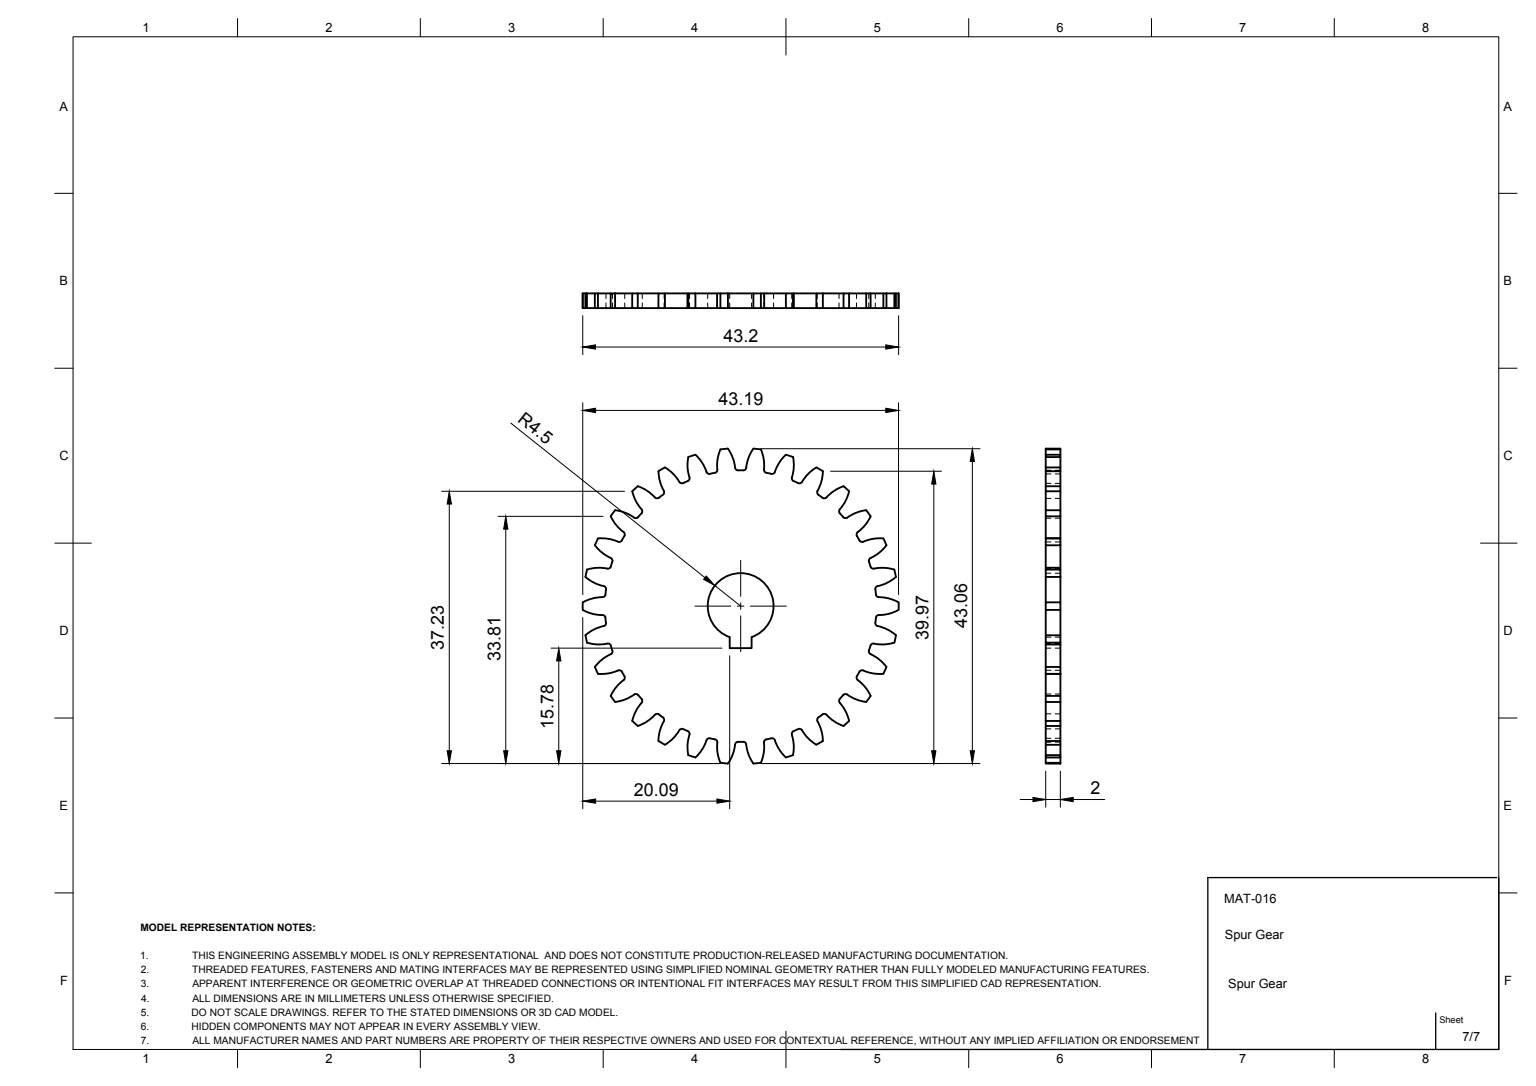
ISO-10303-21;
HEADER;
/* Generated by software containing ST-Developer
 * from STEP Tools, Inc. (www.steptools.com) 
 */

FILE_DESCRIPTION(
/* description */ ('STEP AP214'),
/* implementation_level */ '2;1');

FILE_NAME(
/* name */ 'Spur Gear.step',
/* time_stamp */ '2026-11-14T06:10:26-08:00',
/* author */ (''),
/* organization */ (''),
/* preprocessor_version */ 'ST-DEVELOPER v20.2',
/* originating_system */ 'Autodesk Translation Framework v15.17.0.0',
/* authorisation */ '');

FILE_SCHEMA (('AUTOMOTIVE_DESIGN { 1 0 10303 214 3 1 1 }'));
ENDSEC;

DATA;
#10=MECHANICAL_DESIGN_GEOMETRIC_PRESENTATION_REPRESENTATION('',(#166),#10413);
#150=SHAPE_REPRESENTATION_RELATIONSHIP('SRR','None',#10455,#158);
#158=ADVANCED_BREP_SHAPE_REPRESENTATION('',(#174),#10407);
#166=STYLED_ITEM('',(#10502),#174);
#174=MANIFOLD_SOLID_BREP('Body1',#5301);
#199=FACE_BOUND('',#668,.T.);
#200=FACE_BOUND('',#670,.T.);
#240=PLANE('',#5611);
#241=PLANE('',#5745);
#242=PLANE('',#6012);
#243=PLANE('',#6013);
#244=PLANE('',#6014);
#310=FACE_OUTER_BOUND('',#619,.T.);
#311=FACE_OUTER_BOUND('',#620,.T.);
#312=FACE_OUTER_BOUND('',#621,.T.);
#313=FACE_OUTER_BOUND('',#622,.T.);
#314=FACE_OUTER_BOUND('',#623,.T.);
#315=FACE_OUTER_BOUND('',#624,.T.);
#316=FACE_OUTER_BOUND('',#625,.T.);
#317=FACE_OUTER_BOUND('',#626,.T.);
#318=FACE_OUTER_BOUND('',#627,.T.);
#319=FACE_OUTER_BOUND('',#628,.T.);
#320=FACE_OUTER_BOUND('',#629,.T.);
#321=FACE_OUTER_BOUND('',#630,.T.);
#322=FACE_OUTER_BOUND('',#631,.T.);
#323=FACE_OUTER_BOUND('',#632,.T.);
#324=FACE_OUTER_BOUND('',#633,.T.);
#325=FACE_OUTER_BOUND('',#634,.T.);
#326=FACE_OUTER_BOUND('',#635,.T.);
#327=FACE_OUTER_BOUND('',#636,.T.);
#328=FACE_OUTER_BOUND('',#637,.T.);
#329=FACE_OUTER_BOUND('',#638,.T.);
#330=FACE_OUTER_BOUND('',#639,.T.);
#331=FACE_OUTER_BOUND('',#640,.T.);
#332=FACE_OUTER_BOUND('',#641,.T.);
#333=FACE_OUTER_BOUND('',#642,.T.);
#334=FACE_OUTER_BOUND('',#643,.T.);
#335=FACE_OUTER_BOUND('',#644,.T.);
#336=FACE_OUTER_BOUND('',#645,.T.);
#337=FACE_OUTER_BOUND('',#646,.T.);
#338=FACE_OUTER_BOUND('',#647,.T.);
#339=FACE_OUTER_BOUND('',#648,.T.);
#340=FACE_OUTER_BOUND('',#649,.T.);
#341=FACE_OUTER_BOUND('',#650,.T.);
#342=FACE_OUTER_BOUND('',#651,.T.);
#343=FACE_OUTER_BOUND('',#652,.T.);
#344=FACE_OUTER_BOUND('',#653,.T.);
#345=FACE_OUTER_BOUND('',#654,.T.);
#346=FACE_OUTER_BOUND('',#655,.T.);
#347=FACE_OUTER_BOUND('',#656,.T.);
#348=FACE_OUTER_BOUND('',#657,.T.);
#349=FACE_OUTER_BOUND('',#658,.T.);
#350=FACE_OUTER_BOUND('',#659,.T.);
#351=FACE_OUTER_BOUND('',#660,.T.);
#352=FACE_OUTER_BOUND('',#661,.T.);
#353=FACE_OUTER_BOUND('',#662,.T.);
#354=FACE_OUTER_BOUND('',#663,.T.);
#355=FACE_OUTER_BOUND('',#664,.T.);
#356=FACE_OUTER_BOUND('',#665,.T.);
#357=FACE_OUTER_BOUND('',#666,.T.);
#358=FACE_OUTER_BOUND('',#667,.T.);
#359=FACE_OUTER_BOUND('',#669,.T.);
#360=FACE_OUTER_BOUND('',#671,.T.);
#361=FACE_OUTER_BOUND('',#672,.T.);
#362=FACE_OUTER_BOUND('',#673,.T.);
#363=FACE_OUTER_BOUND('',#674,.T.);
#364=FACE_OUTER_BOUND('',#675,.T.);
#365=FACE_OUTER_BOUND('',#676,.T.);
#366=FACE_OUTER_BOUND('',#677,.T.);
#367=FACE_OUTER_BOUND('',#678,.T.);
#368=FACE_OUTER_BOUND('',#679,.T.);
#369=FACE_OUTER_BOUND('',#680,.T.);
#370=FACE_OUTER_BOUND('',#681,.T.);
#371=FACE_OUTER_BOUND('',#682,.T.);
#372=FACE_OUTER_BOUND('',#683,.T.);
#373=FACE_OUTER_BOUND('',#684,.T.);
#374=FACE_OUTER_BOUND('',#685,.T.);
#375=FACE_OUTER_BOUND('',#686,.T.);
#376=FACE_OUTER_BOUND('',#687,.T.);
#377=FACE_OUTER_BOUND('',#688,.T.);
#378=FACE_OUTER_BOUND('',#689,.T.);
#379=FACE_OUTER_BOUND('',#690,.T.);
#380=FACE_OUTER_BOUND('',#691,.T.);
#381=FACE_OUTER_BOUND('',#692,.T.);
#382=FACE_OUTER_BOUND('',#693,.T.);
#383=FACE_OUTER_BOUND('',#694,.T.);
#384=FACE_OUTER_BOUND('',#695,.T.);
#385=FACE_OUTER_BOUND('',#696,.T.);
#386=FACE_OUTER_BOUND('',#697,.T.);
#387=FACE_OUTER_BOUND('',#698,.T.);
#388=FACE_OUTER_BOUND('',#699,.T.);
#389=FACE_OUTER_BOUND('',#700,.T.);
#390=FACE_OUTER_BOUND('',#701,.T.);
#391=FACE_OUTER_BOUND('',#702,.T.);
#392=FACE_OUTER_BOUND('',#703,.T.);
#393=FACE_OUTER_BOUND('',#704,.T.);
#394=FACE_OUTER_BOUND('',#705,.T.);
#395=FACE_OUTER_BOUND('',#706,.T.);
#396=FACE_OUTER_BOUND('',#707,.T.);
#397=FACE_OUTER_BOUND('',#708,.T.);
#398=FACE_OUTER_BOUND('',#709,.T.);
#399=FACE_OUTER_BOUND('',#710,.T.);
#400=FACE_OUTER_BOUND('',#711,.T.);
#401=FACE_OUTER_BOUND('',#712,.T.);
#402=FACE_OUTER_BOUND('',#713,.T.);
#403=FACE_OUTER_BOUND('',#714,.T.);
#404=FACE_OUTER_BOUND('',#715,.T.);
#405=FACE_OUTER_BOUND('',#716,.T.);
#406=FACE_OUTER_BOUND('',#717,.T.);
#407=FACE_OUTER_BOUND('',#718,.T.);
#408=FACE_OUTER_BOUND('',#719,.T.);
#409=FACE_OUTER_BOUND('',#720,.T.);
#410=FACE_OUTER_BOUND('',#721,.T.);
#411=FACE_OUTER_BOUND('',#722,.T.);
#412=FACE_OUTER_BOUND('',#723,.T.);
#413=FACE_OUTER_BOUND('',#724,.T.);
#414=FACE_OUTER_BOUND('',#725,.T.);
#415=FACE_OUTER_BOUND('',#726,.T.);
#416=FACE_OUTER_BOUND('',#727,.T.);
#417=FACE_OUTER_BOUND('',#728,.T.);
#418=FACE_OUTER_BOUND('',#729,.T.);
#419=FACE_OUTER_BOUND('',#730,.T.);
#420=FACE_OUTER_BOUND('',#731,.T.);
#421=FACE_OUTER_BOUND('',#732,.T.);
#422=FACE_OUTER_BOUND('',#733,.T.);
#423=FACE_OUTER_BOUND('',#734,.T.);
#424=FACE_OUTER_BOUND('',#735,.T.);
#425=FACE_OUTER_BOUND('',#736,.T.);
#426=FACE_OUTER_BOUND('',#737,.T.);
#427=FACE_OUTER_BOUND('',#738,.T.);
#428=FACE_OUTER_BOUND('',#739,.T.);
#429=FACE_OUTER_BOUND('',#740,.T.);
#430=FACE_OUTER_BOUND('',#741,.T.);
#431=FACE_OUTER_BOUND('',#742,.T.);
#432=FACE_OUTER_BOUND('',#743,.T.);
#433=FACE_OUTER_BOUND('',#744,.T.);
#434=FACE_OUTER_BOUND('',#745,.T.);
#435=FACE_OUTER_BOUND('',#746,.T.);
#436=FACE_OUTER_BOUND('',#747,.T.);
#437=FACE_OUTER_BOUND('',#748,.T.);
#438=FACE_OUTER_BOUND('',#749,.T.);
#439=FACE_OUTER_BOUND('',#750,.T.);
#440=FACE_OUTER_BOUND('',#751,.T.);
#441=FACE_OUTER_BOUND('',#752,.T.);
#442=FACE_OUTER_BOUND('',#753,.T.);
#443=FACE_OUTER_BOUND('',#754,.T.);
#444=FACE_OUTER_BOUND('',#755,.T.);
#445=FACE_OUTER_BOUND('',#756,.T.);
#446=FACE_OUTER_BOUND('',#757,.T.);
#447=FACE_OUTER_BOUND('',#758,.T.);
#448=FACE_OUTER_BOUND('',#759,.T.);
#449=FACE_OUTER_BOUND('',#760,.T.);
#450=FACE_OUTER_BOUND('',#761,.T.);
#451=FACE_OUTER_BOUND('',#762,.T.);
#452=FACE_OUTER_BOUND('',#763,.T.);
#453=FACE_OUTER_BOUND('',#764,.T.);
#454=FACE_OUTER_BOUND('',#765,.T.);
#455=FACE_OUTER_BOUND('',#766,.T.);
#456=FACE_OUTER_BOUND('',#767,.T.);
#457=FACE_OUTER_BOUND('',#768,.T.);
#458=FACE_OUTER_BOUND('',#769,.T.);
#459=FACE_OUTER_BOUND('',#770,.T.);
#460=FACE_OUTER_BOUND('',#771,.T.);
#461=FACE_OUTER_BOUND('',#772,.T.);
#462=FACE_OUTER_BOUND('',#773,.T.);
#463=FACE_OUTER_BOUND('',#774,.T.);
#464=FACE_OUTER_BOUND('',#775,.T.);
#465=FACE_OUTER_BOUND('',#776,.T.);
#466=FACE_OUTER_BOUND('',#777,.T.);
#467=FACE_OUTER_BOUND('',#778,.T.);
#468=FACE_OUTER_BOUND('',#779,.T.);
#469=FACE_OUTER_BOUND('',#780,.T.);
#470=FACE_OUTER_BOUND('',#781,.T.);
#471=FACE_OUTER_BOUND('',#782,.T.);
#472=FACE_OUTER_BOUND('',#783,.T.);
#473=FACE_OUTER_BOUND('',#784,.T.);
#474=FACE_OUTER_BOUND('',#785,.T.);
#475=FACE_OUTER_BOUND('',#786,.T.);
#476=FACE_OUTER_BOUND('',#787,.T.);
#477=FACE_OUTER_BOUND('',#788,.T.);
#478=FACE_OUTER_BOUND('',#789,.T.);
#479=FACE_OUTER_BOUND('',#790,.T.);
#480=FACE_OUTER_BOUND('',#791,.T.);
#481=FACE_OUTER_BOUND('',#792,.T.);
#482=FACE_OUTER_BOUND('',#793,.T.);
#483=FACE_OUTER_BOUND('',#794,.T.);
#484=FACE_OUTER_BOUND('',#795,.T.);
#485=FACE_OUTER_BOUND('',#796,.T.);
#486=FACE_OUTER_BOUND('',#797,.T.);
#487=FACE_OUTER_BOUND('',#798,.T.);
#488=FACE_OUTER_BOUND('',#799,.T.);
#489=FACE_OUTER_BOUND('',#800,.T.);
#490=FACE_OUTER_BOUND('',#801,.T.);
#491=FACE_OUTER_BOUND('',#802,.T.);
#492=FACE_OUTER_BOUND('',#803,.T.);
#493=FACE_OUTER_BOUND('',#804,.T.);
#494=FACE_OUTER_BOUND('',#805,.T.);
#495=FACE_OUTER_BOUND('',#806,.T.);
#619=EDGE_LOOP('',(#3374,#3375,#3376,#3377));
#620=EDGE_LOOP('',(#3378,#3379,#3380,#3381));
#621=EDGE_LOOP('',(#3382,#3383,#3384,#3385));
#622=EDGE_LOOP('',(#3386,#3387,#3388,#3389));
#623=EDGE_LOOP('',(#3390,#3391,#3392,#3393));
#624=EDGE_LOOP('',(#3394,#3395,#3396,#3397));
#625=EDGE_LOOP('',(#3398,#3399,#3400,#3401));
#626=EDGE_LOOP('',(#3402,#3403,#3404,#3405));
#627=EDGE_LOOP('',(#3406,#3407,#3408,#3409));
#628=EDGE_LOOP('',(#3410,#3411,#3412,#3413));
#629=EDGE_LOOP('',(#3414,#3415,#3416,#3417));
#630=EDGE_LOOP('',(#3418,#3419,#3420,#3421));
#631=EDGE_LOOP('',(#3422,#3423,#3424,#3425));
#632=EDGE_LOOP('',(#3426,#3427,#3428,#3429));
#633=EDGE_LOOP('',(#3430,#3431,#3432,#3433));
#634=EDGE_LOOP('',(#3434,#3435,#3436,#3437));
#635=EDGE_LOOP('',(#3438,#3439,#3440,#3441));
#636=EDGE_LOOP('',(#3442,#3443,#3444,#3445));
#637=EDGE_LOOP('',(#3446,#3447,#3448,#3449));
#638=EDGE_LOOP('',(#3450,#3451,#3452,#3453));
#639=EDGE_LOOP('',(#3454,#3455,#3456,#3457));
#640=EDGE_LOOP('',(#3458,#3459,#3460,#3461));
#641=EDGE_LOOP('',(#3462,#3463,#3464,#3465));
#642=EDGE_LOOP('',(#3466,#3467,#3468,#3469));
#643=EDGE_LOOP('',(#3470,#3471,#3472,#3473));
#644=EDGE_LOOP('',(#3474,#3475,#3476,#3477));
#645=EDGE_LOOP('',(#3478,#3479,#3480,#3481));
#646=EDGE_LOOP('',(#3482,#3483,#3484,#3485));
#647=EDGE_LOOP('',(#3486,#3487,#3488,#3489));
#648=EDGE_LOOP('',(#3490,#3491,#3492,#3493));
#649=EDGE_LOOP('',(#3494,#3495,#3496,#3497));
#650=EDGE_LOOP('',(#3498,#3499,#3500,#3501));
#651=EDGE_LOOP('',(#3502,#3503,#3504,#3505));
#652=EDGE_LOOP('',(#3506,#3507,#3508,#3509));
#653=EDGE_LOOP('',(#3510,#3511,#3512,#3513));
#654=EDGE_LOOP('',(#3514,#3515,#3516,#3517));
#655=EDGE_LOOP('',(#3518,#3519,#3520,#3521));
#656=EDGE_LOOP('',(#3522,#3523,#3524,#3525));
#657=EDGE_LOOP('',(#3526,#3527,#3528,#3529));
#658=EDGE_LOOP('',(#3530,#3531,#3532,#3533));
#659=EDGE_LOOP('',(#3534,#3535,#3536,#3537));
#660=EDGE_LOOP('',(#3538,#3539,#3540,#3541));
#661=EDGE_LOOP('',(#3542,#3543,#3544,#3545));
#662=EDGE_LOOP('',(#3546,#3547,#3548,#3549));
#663=EDGE_LOOP('',(#3550,#3551,#3552,#3553));
#664=EDGE_LOOP('',(#3554,#3555,#3556,#3557));
#665=EDGE_LOOP('',(#3558,#3559,#3560,#3561));
#666=EDGE_LOOP('',(#3562,#3563,#3564,#3565));
#667=EDGE_LOOP('',(#3566,#3567,#3568,#3569,#3570,#3571,#3572,#3573,#3574,
#3575,#3576,#3577,#3578,#3579,#3580,#3581,#3582,#3583,#3584,#3585,#3586,
#3587,#3588,#3589,#3590,#3591,#3592,#3593,#3594,#3595,#3596,#3597,#3598,
#3599,#3600,#3601,#3602,#3603,#3604,#3605,#3606,#3607,#3608,#3609,#3610,
#3611,#3612,#3613,#3614,#3615,#3616,#3617,#3618,#3619,#3620,#3621,#3622,
#3623,#3624,#3625,#3626,#3627,#3628,#3629,#3630,#3631,#3632,#3633,#3634,
#3635,#3636,#3637,#3638,#3639,#3640,#3641,#3642,#3643,#3644,#3645,#3646,
#3647,#3648,#3649,#3650,#3651,#3652,#3653,#3654,#3655,#3656,#3657,#3658,
#3659,#3660,#3661,#3662,#3663,#3664,#3665,#3666,#3667,#3668,#3669,#3670,
#3671,#3672,#3673,#3674,#3675,#3676,#3677,#3678,#3679,#3680,#3681,#3682,
#3683,#3684,#3685,#3686,#3687,#3688,#3689,#3690,#3691,#3692,#3693,#3694,
#3695,#3696,#3697,#3698,#3699,#3700,#3701,#3702,#3703,#3704,#3705,#3706,
#3707,#3708,#3709,#3710,#3711,#3712,#3713,#3714,#3715,#3716,#3717,#3718,
#3719,#3720,#3721,#3722,#3723,#3724,#3725,#3726,#3727,#3728,#3729,#3730,
#3731,#3732,#3733,#3734,#3735,#3736,#3737,#3738,#3739,#3740,#3741,#3742,
#3743,#3744,#3745));
#668=EDGE_LOOP('',(#3746,#3747,#3748,#3749));
#669=EDGE_LOOP('',(#3750,#3751,#3752,#3753,#3754,#3755,#3756,#3757,#3758,
#3759,#3760,#3761,#3762,#3763,#3764,#3765,#3766,#3767,#3768,#3769,#3770,
#3771,#3772,#3773,#3774,#3775,#3776,#3777,#3778,#3779,#3780,#3781,#3782,
#3783,#3784,#3785,#3786,#3787,#3788,#3789,#3790,#3791,#3792,#3793,#3794,
#3795,#3796,#3797,#3798,#3799,#3800,#3801,#3802,#3803,#3804,#3805,#3806,
#3807,#3808,#3809,#3810,#3811,#3812,#3813,#3814,#3815,#3816,#3817,#3818,
#3819,#3820,#3821,#3822,#3823,#3824,#3825,#3826,#3827,#3828,#3829,#3830,
#3831,#3832,#3833,#3834,#3835,#3836,#3837,#3838,#3839,#3840,#3841,#3842,
#3843,#3844,#3845,#3846,#3847,#3848,#3849,#3850,#3851,#3852,#3853,#3854,
#3855,#3856,#3857,#3858,#3859,#3860,#3861,#3862,#3863,#3864,#3865,#3866,
#3867,#3868,#3869,#3870,#3871,#3872,#3873,#3874,#3875,#3876,#3877,#3878,
#3879,#3880,#3881,#3882,#3883,#3884,#3885,#3886,#3887,#3888,#3889,#3890,
#3891,#3892,#3893,#3894,#3895,#3896,#3897,#3898,#3899,#3900,#3901,#3902,
#3903,#3904,#3905,#3906,#3907,#3908,#3909,#3910,#3911,#3912,#3913,#3914,
#3915,#3916,#3917,#3918,#3919,#3920,#3921,#3922,#3923,#3924,#3925,#3926,
#3927,#3928,#3929));
#670=EDGE_LOOP('',(#3930,#3931,#3932,#3933));
#671=EDGE_LOOP('',(#3934,#3935,#3936,#3937));
#672=EDGE_LOOP('',(#3938,#3939,#3940,#3941));
#673=EDGE_LOOP('',(#3942,#3943,#3944,#3945));
#674=EDGE_LOOP('',(#3946,#3947,#3948,#3949));
#675=EDGE_LOOP('',(#3950,#3951,#3952,#3953));
#676=EDGE_LOOP('',(#3954,#3955,#3956,#3957));
#677=EDGE_LOOP('',(#3958,#3959,#3960,#3961));
#678=EDGE_LOOP('',(#3962,#3963,#3964,#3965));
#679=EDGE_LOOP('',(#3966,#3967,#3968,#3969));
#680=EDGE_LOOP('',(#3970,#3971,#3972,#3973));
#681=EDGE_LOOP('',(#3974,#3975,#3976,#3977));
#682=EDGE_LOOP('',(#3978,#3979,#3980,#3981));
#683=EDGE_LOOP('',(#3982,#3983,#3984,#3985));
#684=EDGE_LOOP('',(#3986,#3987,#3988,#3989));
#685=EDGE_LOOP('',(#3990,#3991,#3992,#3993));
#686=EDGE_LOOP('',(#3994,#3995,#3996,#3997));
#687=EDGE_LOOP('',(#3998,#3999,#4000,#4001));
#688=EDGE_LOOP('',(#4002,#4003,#4004,#4005));
#689=EDGE_LOOP('',(#4006,#4007,#4008,#4009));
#690=EDGE_LOOP('',(#4010,#4011,#4012,#4013));
#691=EDGE_LOOP('',(#4014,#4015,#4016,#4017));
#692=EDGE_LOOP('',(#4018,#4019,#4020,#4021));
#693=EDGE_LOOP('',(#4022,#4023,#4024,#4025));
#694=EDGE_LOOP('',(#4026,#4027,#4028,#4029));
#695=EDGE_LOOP('',(#4030,#4031,#4032,#4033));
#696=EDGE_LOOP('',(#4034,#4035,#4036,#4037));
#697=EDGE_LOOP('',(#4038,#4039,#4040,#4041));
#698=EDGE_LOOP('',(#4042,#4043,#4044,#4045));
#699=EDGE_LOOP('',(#4046,#4047,#4048,#4049));
#700=EDGE_LOOP('',(#4050,#4051,#4052,#4053));
#701=EDGE_LOOP('',(#4054,#4055,#4056,#4057));
#702=EDGE_LOOP('',(#4058,#4059,#4060,#4061));
#703=EDGE_LOOP('',(#4062,#4063,#4064,#4065));
#704=EDGE_LOOP('',(#4066,#4067,#4068,#4069));
#705=EDGE_LOOP('',(#4070,#4071,#4072,#4073));
#706=EDGE_LOOP('',(#4074,#4075,#4076,#4077));
#707=EDGE_LOOP('',(#4078,#4079,#4080,#4081));
#708=EDGE_LOOP('',(#4082,#4083,#4084,#4085));
#709=EDGE_LOOP('',(#4086,#4087,#4088,#4089));
#710=EDGE_LOOP('',(#4090,#4091,#4092,#4093));
#711=EDGE_LOOP('',(#4094,#4095,#4096,#4097));
#712=EDGE_LOOP('',(#4098,#4099,#4100,#4101));
#713=EDGE_LOOP('',(#4102,#4103,#4104,#4105));
#714=EDGE_LOOP('',(#4106,#4107,#4108,#4109));
#715=EDGE_LOOP('',(#4110,#4111,#4112,#4113));
#716=EDGE_LOOP('',(#4114,#4115,#4116,#4117));
#717=EDGE_LOOP('',(#4118,#4119,#4120,#4121));
#718=EDGE_LOOP('',(#4122,#4123,#4124,#4125));
#719=EDGE_LOOP('',(#4126,#4127,#4128,#4129));
#720=EDGE_LOOP('',(#4130,#4131,#4132,#4133));
#721=EDGE_LOOP('',(#4134,#4135,#4136,#4137));
#722=EDGE_LOOP('',(#4138,#4139,#4140,#4141));
#723=EDGE_LOOP('',(#4142,#4143,#4144,#4145));
#724=EDGE_LOOP('',(#4146,#4147,#4148,#4149));
#725=EDGE_LOOP('',(#4150,#4151,#4152,#4153));
#726=EDGE_LOOP('',(#4154,#4155,#4156,#4157));
#727=EDGE_LOOP('',(#4158,#4159,#4160,#4161));
#728=EDGE_LOOP('',(#4162,#4163,#4164,#4165));
#729=EDGE_LOOP('',(#4166,#4167,#4168,#4169));
#730=EDGE_LOOP('',(#4170,#4171,#4172,#4173));
#731=EDGE_LOOP('',(#4174,#4175,#4176,#4177));
#732=EDGE_LOOP('',(#4178,#4179,#4180,#4181));
#733=EDGE_LOOP('',(#4182,#4183,#4184,#4185));
#734=EDGE_LOOP('',(#4186,#4187,#4188,#4189));
#735=EDGE_LOOP('',(#4190,#4191,#4192,#4193));
#736=EDGE_LOOP('',(#4194,#4195,#4196,#4197));
#737=EDGE_LOOP('',(#4198,#4199,#4200,#4201));
#738=EDGE_LOOP('',(#4202,#4203,#4204,#4205));
#739=EDGE_LOOP('',(#4206,#4207,#4208,#4209));
#740=EDGE_LOOP('',(#4210,#4211,#4212,#4213));
#741=EDGE_LOOP('',(#4214,#4215,#4216,#4217));
#742=EDGE_LOOP('',(#4218,#4219,#4220,#4221));
#743=EDGE_LOOP('',(#4222,#4223,#4224,#4225));
#744=EDGE_LOOP('',(#4226,#4227,#4228,#4229));
#745=EDGE_LOOP('',(#4230,#4231,#4232,#4233));
#746=EDGE_LOOP('',(#4234,#4235,#4236,#4237));
#747=EDGE_LOOP('',(#4238,#4239,#4240,#4241));
#748=EDGE_LOOP('',(#4242,#4243,#4244,#4245));
#749=EDGE_LOOP('',(#4246,#4247,#4248,#4249));
#750=EDGE_LOOP('',(#4250,#4251,#4252,#4253));
#751=EDGE_LOOP('',(#4254,#4255,#4256,#4257));
#752=EDGE_LOOP('',(#4258,#4259,#4260,#4261));
#753=EDGE_LOOP('',(#4262,#4263,#4264,#4265));
#754=EDGE_LOOP('',(#4266,#4267,#4268,#4269));
#755=EDGE_LOOP('',(#4270,#4271,#4272,#4273));
#756=EDGE_LOOP('',(#4274,#4275,#4276,#4277));
#757=EDGE_LOOP('',(#4278,#4279,#4280,#4281));
#758=EDGE_LOOP('',(#4282,#4283,#4284,#4285));
#759=EDGE_LOOP('',(#4286,#4287,#4288,#4289));
#760=EDGE_LOOP('',(#4290,#4291,#4292,#4293));
#761=EDGE_LOOP('',(#4294,#4295,#4296,#4297));
#762=EDGE_LOOP('',(#4298,#4299,#4300,#4301));
#763=EDGE_LOOP('',(#4302,#4303,#4304,#4305));
#764=EDGE_LOOP('',(#4306,#4307,#4308,#4309));
#765=EDGE_LOOP('',(#4310,#4311,#4312,#4313));
#766=EDGE_LOOP('',(#4314,#4315,#4316,#4317));
#767=EDGE_LOOP('',(#4318,#4319,#4320,#4321));
#768=EDGE_LOOP('',(#4322,#4323,#4324,#4325));
#769=EDGE_LOOP('',(#4326,#4327,#4328,#4329));
#770=EDGE_LOOP('',(#4330,#4331,#4332,#4333));
#771=EDGE_LOOP('',(#4334,#4335,#4336,#4337));
#772=EDGE_LOOP('',(#4338,#4339,#4340,#4341));
#773=EDGE_LOOP('',(#4342,#4343,#4344,#4345));
#774=EDGE_LOOP('',(#4346,#4347,#4348,#4349));
#775=EDGE_LOOP('',(#4350,#4351,#4352,#4353));
#776=EDGE_LOOP('',(#4354,#4355,#4356,#4357));
#777=EDGE_LOOP('',(#4358,#4359,#4360,#4361));
#778=EDGE_LOOP('',(#4362,#4363,#4364,#4365));
#779=EDGE_LOOP('',(#4366,#4367,#4368,#4369));
#780=EDGE_LOOP('',(#4370,#4371,#4372,#4373));
#781=EDGE_LOOP('',(#4374,#4375,#4376,#4377));
#782=EDGE_LOOP('',(#4378,#4379,#4380,#4381));
#783=EDGE_LOOP('',(#4382,#4383,#4384,#4385));
#784=EDGE_LOOP('',(#4386,#4387,#4388,#4389));
#785=EDGE_LOOP('',(#4390,#4391,#4392,#4393));
#786=EDGE_LOOP('',(#4394,#4395,#4396,#4397));
#787=EDGE_LOOP('',(#4398,#4399,#4400,#4401));
#788=EDGE_LOOP('',(#4402,#4403,#4404,#4405));
#789=EDGE_LOOP('',(#4406,#4407,#4408,#4409));
#790=EDGE_LOOP('',(#4410,#4411,#4412,#4413));
#791=EDGE_LOOP('',(#4414,#4415,#4416,#4417));
#792=EDGE_LOOP('',(#4418,#4419,#4420,#4421));
#793=EDGE_LOOP('',(#4422,#4423,#4424,#4425));
#794=EDGE_LOOP('',(#4426,#4427,#4428,#4429));
#795=EDGE_LOOP('',(#4430,#4431,#4432,#4433));
#796=EDGE_LOOP('',(#4434,#4435,#4436,#4437));
#797=EDGE_LOOP('',(#4438,#4439,#4440,#4441));
#798=EDGE_LOOP('',(#4442,#4443,#4444,#4445));
#799=EDGE_LOOP('',(#4446,#4447,#4448,#4449));
#800=EDGE_LOOP('',(#4450,#4451,#4452,#4453));
#801=EDGE_LOOP('',(#4454,#4455,#4456,#4457));
#802=EDGE_LOOP('',(#4458,#4459,#4460,#4461));
#803=EDGE_LOOP('',(#4462,#4463,#4464,#4465));
#804=EDGE_LOOP('',(#4466,#4467,#4468,#4469));
#805=EDGE_LOOP('',(#4470,#4471,#4472,#4473));
#806=EDGE_LOOP('',(#4474,#4475,#4476,#4477));
#938=LINE('',#8119,#1229);
#939=LINE('',#8122,#1230);
#940=LINE('',#8128,#1231);
#941=LINE('',#8131,#1232);
#942=LINE('',#8136,#1233);
#943=LINE('',#8143,#1234);
#944=LINE('',#8146,#1235);
#945=LINE('',#8151,#1236);
#946=LINE('',#8158,#1237);
#947=LINE('',#8161,#1238);
#948=LINE('',#8167,#1239);
#949=LINE('',#8173,#1240);
#950=LINE('',#8176,#1241);
#951=LINE('',#8182,#1242);
#952=LINE('',#8188,#1243);
#953=LINE('',#8191,#1244);
#954=LINE('',#8197,#1245);
#955=LINE('',#8200,#1246);
#956=LINE('',#8206,#1247);
#957=LINE('',#8209,#1248);
#958=LINE('',#8215,#1249);
#959=LINE('',#8218,#1250);
#960=LINE('',#8224,#1251);
#961=LINE('',#8227,#1252);
#962=LINE('',#8233,#1253);
#963=LINE('',#8236,#1254);
#964=LINE('',#8242,#1255);
#965=LINE('',#8245,#1256);
#966=LINE('',#8251,#1257);
#967=LINE('',#8254,#1258);
#968=LINE('',#8260,#1259);
#969=LINE('',#8263,#1260);
#970=LINE('',#8269,#1261);
#971=LINE('',#8272,#1262);
#972=LINE('',#8278,#1263);
#973=LINE('',#8281,#1264);
#974=LINE('',#8287,#1265);
#975=LINE('',#8290,#1266);
#976=LINE('',#8296,#1267);
#977=LINE('',#8299,#1268);
#978=LINE('',#8305,#1269);
#979=LINE('',#8308,#1270);
#980=LINE('',#8314,#1271);
#981=LINE('',#8317,#1272);
#982=LINE('',#8323,#1273);
#983=LINE('',#8326,#1274);
#984=LINE('',#8332,#1275);
#985=LINE('',#8335,#1276);
#986=LINE('',#8341,#1277);
#987=LINE('',#8344,#1278);
#988=LINE('',#8350,#1279);
#989=LINE('',#8353,#1280);
#990=LINE('',#8359,#1281);
#991=LINE('',#8362,#1282);
#992=LINE('',#8368,#1283);
#993=LINE('',#8371,#1284);
#994=LINE('',#8377,#1285);
#995=LINE('',#8380,#1286);
#996=LINE('',#8386,#1287);
#997=LINE('',#8389,#1288);
#998=LINE('',#8395,#1289);
#999=LINE('',#8398,#1290);
#1000=LINE('',#8403,#1291);
#1001=LINE('',#8409,#1292);
#1002=LINE('',#8415,#1293);
#1003=LINE('',#8422,#1294);
#1004=LINE('',#8425,#1295);
#1005=LINE('',#8431,#1296);
#1006=LINE('',#8434,#1297);
#1007=LINE('',#8440,#1298);
#1008=LINE('',#8443,#1299);
#1009=LINE('',#8449,#1300);
#1010=LINE('',#8452,#1301);
#1011=LINE('',#8458,#1302);
#1012=LINE('',#8461,#1303);
#1013=LINE('',#8467,#1304);
#1014=LINE('',#8470,#1305);
#1015=LINE('',#8476,#1306);
#1016=LINE('',#8479,#1307);
#1017=LINE('',#8485,#1308);
#1018=LINE('',#8488,#1309);
#1019=LINE('',#8494,#1310);
#1020=LINE('',#8497,#1311);
#1021=LINE('',#8503,#1312);
#1022=LINE('',#8506,#1313);
#1023=LINE('',#8512,#1314);
#1024=LINE('',#8515,#1315);
#1025=LINE('',#8521,#1316);
#1026=LINE('',#8524,#1317);
#1027=LINE('',#8754,#1318);
#1028=LINE('',#8755,#1319);
#1029=LINE('',#8756,#1320);
#1030=LINE('',#8985,#1321);
#1031=LINE('',#8987,#1322);
#1032=LINE('',#8988,#1323);
#1033=LINE('',#8990,#1324);
#1034=LINE('',#8992,#1325);
#1035=LINE('',#8994,#1326);
#1036=LINE('',#8996,#1327);
#1037=LINE('',#8997,#1328);
#1038=LINE('',#9001,#1329);
#1039=LINE('',#9003,#1330);
#1040=LINE('',#9005,#1331);
#1041=LINE('',#9007,#1332);
#1042=LINE('',#9011,#1333);
#1043=LINE('',#9013,#1334);
#1044=LINE('',#9017,#1335);
#1045=LINE('',#9019,#1336);
#1046=LINE('',#9023,#1337);
#1047=LINE('',#9025,#1338);
#1048=LINE('',#9029,#1339);
#1049=LINE('',#9031,#1340);
#1050=LINE('',#9035,#1341);
#1051=LINE('',#9037,#1342);
#1052=LINE('',#9040,#1343);
#1053=LINE('',#9043,#1344);
#1054=LINE('',#9046,#1345);
#1055=LINE('',#9049,#1346);
#1056=LINE('',#9052,#1347);
#1057=LINE('',#9055,#1348);
#1058=LINE('',#9058,#1349);
#1059=LINE('',#9061,#1350);
#1060=LINE('',#9064,#1351);
#1061=LINE('',#9067,#1352);
#1062=LINE('',#9070,#1353);
#1063=LINE('',#9072,#1354);
#1064=LINE('',#9075,#1355);
#1065=LINE('',#9077,#1356);
#1066=LINE('',#9080,#1357);
#1067=LINE('',#9082,#1358);
#1068=LINE('',#9085,#1359);
#1069=LINE('',#9087,#1360);
#1070=LINE('',#9090,#1361);
#1071=LINE('',#9092,#1362);
#1072=LINE('',#9094,#1363);
#1073=LINE('',#9096,#1364);
#1074=LINE('',#9099,#1365);
#1075=LINE('',#9101,#1366);
#1076=LINE('',#9103,#1367);
#1077=LINE('',#9105,#1368);
#1078=LINE('',#9108,#1369);
#1079=LINE('',#9110,#1370);
#1080=LINE('',#9112,#1371);
#1081=LINE('',#9114,#1372);
#1082=LINE('',#9117,#1373);
#1083=LINE('',#9119,#1374);
#1084=LINE('',#9121,#1375);
#1085=LINE('',#9123,#1376);
#1086=LINE('',#9126,#1377);
#1087=LINE('',#9128,#1378);
#1088=LINE('',#9130,#1379);
#1089=LINE('',#9132,#1380);
#1090=LINE('',#9135,#1381);
#1091=LINE('',#9137,#1382);
#1092=LINE('',#9139,#1383);
#1093=LINE('',#9141,#1384);
#1094=LINE('',#9144,#1385);
#1095=LINE('',#9146,#1386);
#1096=LINE('',#9148,#1387);
#1097=LINE('',#9150,#1388);
#1098=LINE('',#9153,#1389);
#1099=LINE('',#9155,#1390);
#1100=LINE('',#9157,#1391);
#1101=LINE('',#9159,#1392);
#1102=LINE('',#9162,#1393);
#1103=LINE('',#9164,#1394);
#1104=LINE('',#9166,#1395);
#1105=LINE('',#9168,#1396);
#1106=LINE('',#9171,#1397);
#1107=LINE('',#9173,#1398);
#1108=LINE('',#9175,#1399);
#1109=LINE('',#9177,#1400);
#1110=LINE('',#9180,#1401);
#1111=LINE('',#9182,#1402);
#1112=LINE('',#9184,#1403);
#1113=LINE('',#9186,#1404);
#1114=LINE('',#9189,#1405);
#1115=LINE('',#9191,#1406);
#1116=LINE('',#9193,#1407);
#1117=LINE('',#9195,#1408);
#1118=LINE('',#9198,#1409);
#1119=LINE('',#9200,#1410);
#1120=LINE('',#9202,#1411);
#1121=LINE('',#9204,#1412);
#1122=LINE('',#9207,#1413);
#1123=LINE('',#9209,#1414);
#1124=LINE('',#9211,#1415);
#1125=LINE('',#9213,#1416);
#1126=LINE('',#9216,#1417);
#1127=LINE('',#9217,#1418);
#1229=VECTOR('',#6340,1000.);
#1230=VECTOR('',#6343,1000.);
#1231=VECTOR('',#6348,1000.);
#1232=VECTOR('',#6351,1000.);
#1233=VECTOR('',#6356,1000.);
#1234=VECTOR('',#6363,1000.);
#1235=VECTOR('',#6366,1000.);
#1236=VECTOR('',#6371,1000.);
#1237=VECTOR('',#6378,1000.);
#1238=VECTOR('',#6381,1000.);
#1239=VECTOR('',#6388,1000.);
#1240=VECTOR('',#6393,1000.);
#1241=VECTOR('',#6396,1000.);
#1242=VECTOR('',#6403,1000.);
#1243=VECTOR('',#6408,1000.);
#1244=VECTOR('',#6411,1000.);
#1245=VECTOR('',#6416,1000.);
#1246=VECTOR('',#6419,1000.);
#1247=VECTOR('',#6424,1000.);
#1248=VECTOR('',#6427,1000.);
#1249=VECTOR('',#6432,1000.);
#1250=VECTOR('',#6435,1000.);
#1251=VECTOR('',#6440,1000.);
#1252=VECTOR('',#6443,1000.);
#1253=VECTOR('',#6448,1000.);
#1254=VECTOR('',#6451,1000.);
#1255=VECTOR('',#6456,1000.);
#1256=VECTOR('',#6459,1000.);
#1257=VECTOR('',#6464,1000.);
#1258=VECTOR('',#6467,1000.);
#1259=VECTOR('',#6472,1000.);
#1260=VECTOR('',#6475,1000.);
#1261=VECTOR('',#6480,1000.);
#1262=VECTOR('',#6483,1000.);
#1263=VECTOR('',#6488,1000.);
#1264=VECTOR('',#6491,1000.);
#1265=VECTOR('',#6496,1000.);
#1266=VECTOR('',#6499,1000.);
#1267=VECTOR('',#6504,1000.);
#1268=VECTOR('',#6507,1000.);
#1269=VECTOR('',#6512,1000.);
#1270=VECTOR('',#6515,1000.);
#1271=VECTOR('',#6520,1000.);
#1272=VECTOR('',#6523,1000.);
#1273=VECTOR('',#6528,1000.);
#1274=VECTOR('',#6531,1000.);
#1275=VECTOR('',#6536,1000.);
#1276=VECTOR('',#6539,1000.);
#1277=VECTOR('',#6544,1000.);
#1278=VECTOR('',#6547,1000.);
#1279=VECTOR('',#6552,1000.);
#1280=VECTOR('',#6555,1000.);
#1281=VECTOR('',#6560,1000.);
#1282=VECTOR('',#6563,1000.);
#1283=VECTOR('',#6568,1000.);
#1284=VECTOR('',#6571,1000.);
#1285=VECTOR('',#6576,1000.);
#1286=VECTOR('',#6579,1000.);
#1287=VECTOR('',#6584,1000.);
#1288=VECTOR('',#6587,1000.);
#1289=VECTOR('',#6592,1000.);
#1290=VECTOR('',#6595,1000.);
#1291=VECTOR('',#6600,1000.);
#1292=VECTOR('',#6607,1000.);
#1293=VECTOR('',#6614,1000.);
#1294=VECTOR('',#6621,1000.);
#1295=VECTOR('',#6624,1000.);
#1296=VECTOR('',#6629,1000.);
#1297=VECTOR('',#6632,1000.);
#1298=VECTOR('',#6637,1000.);
#1299=VECTOR('',#6640,1000.);
#1300=VECTOR('',#6645,1000.);
#1301=VECTOR('',#6648,1000.);
#1302=VECTOR('',#6653,1000.);
#1303=VECTOR('',#6656,1000.);
#1304=VECTOR('',#6661,1000.);
#1305=VECTOR('',#6664,1000.);
#1306=VECTOR('',#6669,1000.);
#1307=VECTOR('',#6672,1000.);
#1308=VECTOR('',#6677,1000.);
#1309=VECTOR('',#6680,1000.);
#1310=VECTOR('',#6685,1000.);
#1311=VECTOR('',#6688,1000.);
#1312=VECTOR('',#6693,1000.);
#1313=VECTOR('',#6696,1000.);
#1314=VECTOR('',#6701,1000.);
#1315=VECTOR('',#6704,1000.);
#1316=VECTOR('',#6709,1000.);
#1317=VECTOR('',#6712,1000.);
#1318=VECTOR('',#6981,1000.);
#1319=VECTOR('',#6982,1000.);
#1320=VECTOR('',#6983,1000.);
#1321=VECTOR('',#7252,1000.);
#1322=VECTOR('',#7253,1000.);
#1323=VECTOR('',#7254,1000.);
#1324=VECTOR('',#7257,1000.);
#1325=VECTOR('',#7260,1000.);
#1326=VECTOR('',#7263,1000.);
#1327=VECTOR('',#7266,1000.);
#1328=VECTOR('',#7267,1000.);
#1329=VECTOR('',#7274,1000.);
#1330=VECTOR('',#7277,1000.);
#1331=VECTOR('',#7280,1000.);
#1332=VECTOR('',#7283,1000.);
#1333=VECTOR('',#7290,1000.);
#1334=VECTOR('',#7293,1000.);
#1335=VECTOR('',#7300,1000.);
#1336=VECTOR('',#7303,1000.);
#1337=VECTOR('',#7310,1000.);
#1338=VECTOR('',#7313,1000.);
#1339=VECTOR('',#7320,1000.);
#1340=VECTOR('',#7323,1000.);
#1341=VECTOR('',#7330,1000.);
#1342=VECTOR('',#7333,1000.);
#1343=VECTOR('',#7338,1000.);
#1344=VECTOR('',#7343,1000.);
#1345=VECTOR('',#7348,1000.);
#1346=VECTOR('',#7353,1000.);
#1347=VECTOR('',#7358,1000.);
#1348=VECTOR('',#7363,1000.);
#1349=VECTOR('',#7368,1000.);
#1350=VECTOR('',#7373,1000.);
#1351=VECTOR('',#7378,1000.);
#1352=VECTOR('',#7383,1000.);
#1353=VECTOR('',#7388,1000.);
#1354=VECTOR('',#7391,1000.);
#1355=VECTOR('',#7396,1000.);
#1356=VECTOR('',#7399,1000.);
#1357=VECTOR('',#7404,1000.);
#1358=VECTOR('',#7407,1000.);
#1359=VECTOR('',#7412,1000.);
#1360=VECTOR('',#7415,1000.);
#1361=VECTOR('',#7420,1000.);
#1362=VECTOR('',#7423,1000.);
#1363=VECTOR('',#7426,1000.);
#1364=VECTOR('',#7429,1000.);
#1365=VECTOR('',#7434,1000.);
#1366=VECTOR('',#7437,1000.);
#1367=VECTOR('',#7440,1000.);
#1368=VECTOR('',#7443,1000.);
#1369=VECTOR('',#7448,1000.);
#1370=VECTOR('',#7451,1000.);
#1371=VECTOR('',#7454,1000.);
#1372=VECTOR('',#7457,1000.);
#1373=VECTOR('',#7462,1000.);
#1374=VECTOR('',#7465,1000.);
#1375=VECTOR('',#7468,1000.);
#1376=VECTOR('',#7471,1000.);
#1377=VECTOR('',#7476,1000.);
#1378=VECTOR('',#7479,1000.);
#1379=VECTOR('',#7482,1000.);
#1380=VECTOR('',#7485,1000.);
#1381=VECTOR('',#7490,1000.);
#1382=VECTOR('',#7493,1000.);
#1383=VECTOR('',#7496,1000.);
#1384=VECTOR('',#7499,1000.);
#1385=VECTOR('',#7504,1000.);
#1386=VECTOR('',#7507,1000.);
#1387=VECTOR('',#7510,1000.);
#1388=VECTOR('',#7513,1000.);
#1389=VECTOR('',#7518,1000.);
#1390=VECTOR('',#7521,1000.);
#1391=VECTOR('',#7524,1000.);
#1392=VECTOR('',#7527,1000.);
#1393=VECTOR('',#7532,1000.);
#1394=VECTOR('',#7535,1000.);
#1395=VECTOR('',#7538,1000.);
#1396=VECTOR('',#7541,1000.);
#1397=VECTOR('',#7546,1000.);
#1398=VECTOR('',#7549,1000.);
#1399=VECTOR('',#7552,1000.);
#1400=VECTOR('',#7555,1000.);
#1401=VECTOR('',#7560,1000.);
#1402=VECTOR('',#7563,1000.);
#1403=VECTOR('',#7566,1000.);
#1404=VECTOR('',#7569,1000.);
#1405=VECTOR('',#7574,1000.);
#1406=VECTOR('',#7577,1000.);
#1407=VECTOR('',#7580,1000.);
#1408=VECTOR('',#7583,1000.);
#1409=VECTOR('',#7588,1000.);
#1410=VECTOR('',#7591,1000.);
#1411=VECTOR('',#7594,1000.);
#1412=VECTOR('',#7597,1000.);
#1413=VECTOR('',#7602,1000.);
#1414=VECTOR('',#7605,1000.);
#1415=VECTOR('',#7608,1000.);
#1416=VECTOR('',#7611,1000.);
#1417=VECTOR('',#7616,1000.);
#1418=VECTOR('',#7617,1000.);
#1508=CIRCLE('',#5468,4.5);
#1509=CIRCLE('',#5469,4.5);
#1510=CIRCLE('',#5471,0.405000000000006);
#1511=CIRCLE('',#5472,0.405000000000006);
#1512=CIRCLE('',#5474,5.53127226019911);
#1513=CIRCLE('',#5475,5.53127226019911);
#1514=CIRCLE('',#5477,0.404999999999998);
#1515=CIRCLE('',#5478,0.404999999999998);
#1516=CIRCLE('',#5480,5.53127226019911);
#1517=CIRCLE('',#5481,5.53127226019914);
#1518=CIRCLE('',#5483,0.404999999999992);
#1519=CIRCLE('',#5484,0.404999999999992);
#1520=CIRCLE('',#5486,5.53127226019909);
#1521=CIRCLE('',#5487,5.5312722601991);
#1522=CIRCLE('',#5489,0.405);
#1523=CIRCLE('',#5490,0.404999999999998);
#1524=CIRCLE('',#5492,5.53127226019911);
#1525=CIRCLE('',#5493,5.53127226019911);
#1526=CIRCLE('',#5495,0.404999999999999);
#1527=CIRCLE('',#5496,0.404999999999999);
#1528=CIRCLE('',#5498,0.405000000000004);
#1529=CIRCLE('',#5499,0.405000000000003);
#1530=CIRCLE('',#5501,0.405000000000003);
#1531=CIRCLE('',#5502,0.404999999999999);
#1532=CIRCLE('',#5504,0.404999999999999);
#1533=CIRCLE('',#5505,0.404999999999999);
#1534=CIRCLE('',#5507,0.404999999999999);
#1535=CIRCLE('',#5508,0.404999999999999);
#1536=CIRCLE('',#5510,0.404999999999996);
#1537=CIRCLE('',#5511,0.404999999999996);
#1538=CIRCLE('',#5513,0.40500000000001);
#1539=CIRCLE('',#5514,0.40500000000001);
#1540=CIRCLE('',#5516,0.404999999999996);
#1541=CIRCLE('',#5517,0.405000000000001);
#1542=CIRCLE('',#5519,0.404999999999996);
#1543=CIRCLE('',#5520,0.404999999999996);
#1544=CIRCLE('',#5522,0.404999999999996);
#1545=CIRCLE('',#5523,0.404999999999996);
#1546=CIRCLE('',#5525,21.6000000000069);
#1547=CIRCLE('',#5526,21.5999999999974);
#1548=CIRCLE('',#5528,21.6000000000069);
#1549=CIRCLE('',#5529,21.6000000000079);
#1550=CIRCLE('',#5531,21.6000000000022);
#1551=CIRCLE('',#5532,21.6000000000022);
#1552=CIRCLE('',#5534,21.6000000000017);
#1553=CIRCLE('',#5535,21.6000000000017);
#1554=CIRCLE('',#5537,21.6000000000002);
#1555=CIRCLE('',#5538,21.600000000003);
#1556=CIRCLE('',#5540,21.6000000000047);
#1557=CIRCLE('',#5541,21.6000000000107);
#1558=CIRCLE('',#5543,21.6000000000067);
#1559=CIRCLE('',#5544,21.6000000000066);
#1560=CIRCLE('',#5546,21.6000000000054);
#1561=CIRCLE('',#5547,21.600000000006);
#1562=CIRCLE('',#5549,21.599999999993);
#1563=CIRCLE('',#5550,21.5999999999977);
#1564=CIRCLE('',#5552,21.6000000000103);
#1565=CIRCLE('',#5553,21.6000000000038);
#1566=CIRCLE('',#5555,21.5999999999939);
#1567=CIRCLE('',#5556,21.6000000000019);
#1568=CIRCLE('',#5558,21.6000000000017);
#1569=CIRCLE('',#5559,21.599999999998);
#1570=CIRCLE('',#5561,21.6000000000022);
#1571=CIRCLE('',#5562,21.5999999999987);
#1572=CIRCLE('',#5564,21.6000000000105);
#1573=CIRCLE('',#5565,21.6000000000104);
#1574=CIRCLE('',#5567,21.5999999999996);
#1575=CIRCLE('',#5568,21.6000000000046);
#1576=CIRCLE('',#5570,21.6000000000023);
#1577=CIRCLE('',#5571,21.5999999999979);
#1578=CIRCLE('',#5573,21.5999999999993);
#1579=CIRCLE('',#5574,21.6000000000028);
#1580=CIRCLE('',#5576,21.6000000000016);
#1581=CIRCLE('',#5577,21.6000000000009);
#1582=CIRCLE('',#5579,21.5999999999992);
#1583=CIRCLE('',#5580,21.6000000000034);
#1584=CIRCLE('',#5582,21.6000000000071);
#1585=CIRCLE('',#5583,21.6000000000056);
#1586=CIRCLE('',#5585,21.6000000000013);
#1587=CIRCLE('',#5586,21.600000000004);
#1588=CIRCLE('',#5588,21.6000000000017);
#1589=CIRCLE('',#5589,21.6000000000059);
#1590=CIRCLE('',#5591,21.5999999999972);
#1591=CIRCLE('',#5592,21.5999999999972);
#1592=CIRCLE('',#5594,21.5999999999966);
#1593=CIRCLE('',#5595,21.5999999999966);
#1594=CIRCLE('',#5597,21.599999999999);
#1595=CIRCLE('',#5598,21.6000000000073);
#1596=CIRCLE('',#5600,21.6000000000014);
#1597=CIRCLE('',#5601,21.600000000002);
#1598=CIRCLE('',#5603,21.6000000000059);
#1599=CIRCLE('',#5604,21.6000000000053);
#1600=CIRCLE('',#5606,21.6000000000022);
#1601=CIRCLE('',#5607,21.6000000000035);
#1602=CIRCLE('',#5609,21.599999999998);
#1603=CIRCLE('',#5610,21.599999999998);
#1604=CIRCLE('',#5612,5.53127226019917);
#1605=CIRCLE('',#5613,0.405000000000003);
#1606=CIRCLE('',#5614,18.5624999999987);
#1607=CIRCLE('',#5615,0.404999999999999);
#1608=CIRCLE('',#5616,5.53127226019909);
#1609=CIRCLE('',#5617,5.53127226019908);
#1610=CIRCLE('',#5618,0.404999999999999);
#1611=CIRCLE('',#5619,18.562499999997);
#1612=CIRCLE('',#5620,0.405000000000001);
#1613=CIRCLE('',#5621,5.53127226019913);
#1614=CIRCLE('',#5622,5.5312722601991);
#1615=CIRCLE('',#5623,0.405000000000003);
#1616=CIRCLE('',#5624,18.562500000001);
#1617=CIRCLE('',#5625,0.404999999999999);
#1618=CIRCLE('',#5626,5.53127226019911);
#1619=CIRCLE('',#5627,5.53127226019907);
#1620=CIRCLE('',#5628,0.404999999999999);
#1621=CIRCLE('',#5629,18.5625000000035);
#1622=CIRCLE('',#5630,0.405000000000002);
#1623=CIRCLE('',#5631,5.5312722601991);
#1624=CIRCLE('',#5632,5.53127226019912);
#1625=CIRCLE('',#5633,0.405000000000003);
#1626=CIRCLE('',#5634,18.5624999999966);
#1627=CIRCLE('',#5635,0.404999999999999);
#1628=CIRCLE('',#5636,5.53127226019916);
#1629=CIRCLE('',#5637,5.53127226019916);
#1630=CIRCLE('',#5638,0.405000000000003);
#1631=CIRCLE('',#5639,18.5625000000007);
#1632=CIRCLE('',#5640,0.404999999999999);
#1633=CIRCLE('',#5641,5.53127226019912);
#1634=CIRCLE('',#5642,5.53127226019916);
#1635=CIRCLE('',#5643,0.405000000000003);
#1636=CIRCLE('',#5644,18.5625000000044);
#1637=CIRCLE('',#5645,0.405000000000003);
#1638=CIRCLE('',#5646,5.53127226019909);
#1639=CIRCLE('',#5647,5.53127226019908);
#1640=CIRCLE('',#5648,0.40499999999999);
#1641=CIRCLE('',#5649,18.5625000000143);
#1642=CIRCLE('',#5650,0.405000000000008);
#1643=CIRCLE('',#5651,5.53127226019909);
#1644=CIRCLE('',#5652,5.53127226019913);
#1645=CIRCLE('',#5653,0.404999999999997);
#1646=CIRCLE('',#5654,18.5624999999983);
#1647=CIRCLE('',#5655,0.404999999999996);
#1648=CIRCLE('',#5656,5.53127226019912);
#1649=CIRCLE('',#5657,5.53127226019916);
#1650=CIRCLE('',#5658,0.405000000000005);
#1651=CIRCLE('',#5659,18.5625000000123);
#1652=CIRCLE('',#5660,0.404999999999998);
#1653=CIRCLE('',#5661,5.53127226019912);
#1654=CIRCLE('',#5662,5.53127226019913);
#1655=CIRCLE('',#5663,0.404999999999998);
#1656=CIRCLE('',#5664,18.5625000000065);
#1657=CIRCLE('',#5665,0.405000000000003);
#1658=CIRCLE('',#5666,5.5312722601991);
#1659=CIRCLE('',#5667,5.53127226019913);
#1660=CIRCLE('',#5668,0.404999999999999);
#1661=CIRCLE('',#5669,18.5624999999925);
#1662=CIRCLE('',#5670,0.405000000000004);
#1663=CIRCLE('',#5671,5.53127226019914);
#1664=CIRCLE('',#5672,18.5625000000053);
#1665=CIRCLE('',#5673,0.405000000000001);
#1666=CIRCLE('',#5674,5.53127226019909);
#1667=CIRCLE('',#5675,18.5625000000105);
#1668=CIRCLE('',#5676,0.405000000000001);
#1669=CIRCLE('',#5677,5.53127226019915);
#1670=CIRCLE('',#5678,5.5312722601991);
#1671=CIRCLE('',#5679,18.5624999999963);
#1672=CIRCLE('',#5680,0.405000000000004);
#1673=CIRCLE('',#5681,5.53127226019909);
#1674=CIRCLE('',#5682,5.53127226019909);
#1675=CIRCLE('',#5683,18.5625000000014);
#1676=CIRCLE('',#5684,0.404999999999999);
#1677=CIRCLE('',#5685,5.53127226019901);
#1678=CIRCLE('',#5686,5.53127226019916);
#1679=CIRCLE('',#5687,18.5625000000026);
#1680=CIRCLE('',#5688,0.404999999999999);
#1681=CIRCLE('',#5689,5.53127226019912);
#1682=CIRCLE('',#5690,5.5312722601991);
#1683=CIRCLE('',#5691,18.5625000000025);
#1684=CIRCLE('',#5692,0.405000000000001);
#1685=CIRCLE('',#5693,5.5312722601991);
#1686=CIRCLE('',#5694,5.5312722601991);
#1687=CIRCLE('',#5695,18.5625000000043);
#1688=CIRCLE('',#5696,0.404999999999999);
#1689=CIRCLE('',#5697,5.53127226019912);
#1690=CIRCLE('',#5698,5.5312722601991);
#1691=CIRCLE('',#5699,0.404999999999996);
#1692=CIRCLE('',#5700,18.5625000000115);
#1693=CIRCLE('',#5701,5.53127226019912);
#1694=CIRCLE('',#5702,5.5312722601991);
#1695=CIRCLE('',#5703,0.404999999999992);
#1696=CIRCLE('',#5704,18.5625000000082);
#1697=CIRCLE('',#5705,5.53127226019914);
#1698=CIRCLE('',#5706,5.53127226019908);
#1699=CIRCLE('',#5707,0.404999999999996);
#1700=CIRCLE('',#5708,18.562500000006);
#1701=CIRCLE('',#5709,5.53127226019906);
#1702=CIRCLE('',#5710,5.53127226019913);
#1703=CIRCLE('',#5711,0.405000000000003);
#1704=CIRCLE('',#5712,18.5624999999967);
#1705=CIRCLE('',#5713,5.53127226019909);
#1706=CIRCLE('',#5714,5.53127226019907);
#1707=CIRCLE('',#5715,0.404999999999996);
#1708=CIRCLE('',#5716,18.562499999998);
#1709=CIRCLE('',#5717,5.53127226019909);
#1710=CIRCLE('',#5718,5.53127226019907);
#1711=CIRCLE('',#5719,0.405000000000003);
#1712=CIRCLE('',#5720,18.562500000011);
#1713=CIRCLE('',#5721,5.53127226019915);
#1714=CIRCLE('',#5722,0.405000000000003);
#1715=CIRCLE('',#5723,18.5624999999985);
#1716=CIRCLE('',#5724,21.6000000000043);
#1717=CIRCLE('',#5725,5.53127226019911);
#1718=CIRCLE('',#5726,0.405000000000002);
#1719=CIRCLE('',#5727,18.5625000000073);
#1720=CIRCLE('',#5728,0.404999999999998);
#1721=CIRCLE('',#5729,5.53127226019908);
#1722=CIRCLE('',#5730,5.53127226019911);
#1723=CIRCLE('',#5731,0.404999999999997);
#1724=CIRCLE('',#5732,18.5625000000057);
#1725=CIRCLE('',#5733,0.404999999999998);
#1726=CIRCLE('',#5734,5.53127226019911);
#1727=CIRCLE('',#5735,5.53127226019913);
#1728=CIRCLE('',#5736,0.405000000000003);
#1729=CIRCLE('',#5737,18.56250000001);
#1730=CIRCLE('',#5738,0.404999999999992);
#1731=CIRCLE('',#5739,5.53127226019908);
#1732=CIRCLE('',#5740,5.53127226019912);
#1733=CIRCLE('',#5741,0.404999999999997);
#1734=CIRCLE('',#5742,18.562500000001);
#1735=CIRCLE('',#5743,0.404999999999997);
#1736=CIRCLE('',#5744,5.5312722601991);
#1737=CIRCLE('',#5746,5.53127226019912);
#1738=CIRCLE('',#5747,5.53127226019911);
#1739=CIRCLE('',#5748,0.404999999999996);
#1740=CIRCLE('',#5749,18.562500000001);
#1741=CIRCLE('',#5750,0.405000000000003);
#1742=CIRCLE('',#5751,5.53127226019912);
#1743=CIRCLE('',#5752,5.53127226019908);
#1744=CIRCLE('',#5753,0.404999999999999);
#1745=CIRCLE('',#5754,18.56250000001);
#1746=CIRCLE('',#5755,0.405000000000004);
#1747=CIRCLE('',#5756,5.53127226019912);
#1748=CIRCLE('',#5757,5.5312722601991);
#1749=CIRCLE('',#5758,0.404999999999997);
#1750=CIRCLE('',#5759,18.5625000000057);
#1751=CIRCLE('',#5760,0.404999999999997);
#1752=CIRCLE('',#5761,5.53127226019915);
#1753=CIRCLE('',#5762,5.53127226019911);
#1754=CIRCLE('',#5763,0.404999999999998);
#1755=CIRCLE('',#5764,18.5625000000073);
#1756=CIRCLE('',#5765,0.405000000000002);
#1757=CIRCLE('',#5766,5.5312722601991);
#1758=CIRCLE('',#5767,21.5999999999959);
#1759=CIRCLE('',#5768,18.5624999999985);
#1760=CIRCLE('',#5769,0.405000000000003);
#1761=CIRCLE('',#5770,5.53127226019911);
#1762=CIRCLE('',#5771,18.562500000011);
#1763=CIRCLE('',#5772,0.405000000000003);
#1764=CIRCLE('',#5773,5.53127226019907);
#1765=CIRCLE('',#5774,5.53127226019914);
#1766=CIRCLE('',#5775,18.562499999998);
#1767=CIRCLE('',#5776,0.404999999999996);
#1768=CIRCLE('',#5777,5.53127226019908);
#1769=CIRCLE('',#5778,5.53127226019909);
#1770=CIRCLE('',#5779,18.5624999999967);
#1771=CIRCLE('',#5780,0.405000000000003);
#1772=CIRCLE('',#5781,5.53127226019919);
#1773=CIRCLE('',#5782,5.53127226019911);
#1774=CIRCLE('',#5783,18.562500000006);
#1775=CIRCLE('',#5784,0.404999999999996);
#1776=CIRCLE('',#5785,5.53127226019911);
#1777=CIRCLE('',#5786,5.53127226019915);
#1778=CIRCLE('',#5787,18.5625000000082);
#1779=CIRCLE('',#5788,0.404999999999992);
#1780=CIRCLE('',#5789,5.53127226019912);
#1781=CIRCLE('',#5790,5.53127226019915);
#1782=CIRCLE('',#5791,18.5625000000115);
#1783=CIRCLE('',#5792,0.404999999999996);
#1784=CIRCLE('',#5793,5.53127226019913);
#1785=CIRCLE('',#5794,5.53127226019912);
#1786=CIRCLE('',#5795,0.404999999999999);
#1787=CIRCLE('',#5796,18.5625000000043);
#1788=CIRCLE('',#5797,5.5312722601991);
#1789=CIRCLE('',#5798,5.53127226019909);
#1790=CIRCLE('',#5799,0.405000000000003);
#1791=CIRCLE('',#5800,18.5625000000025);
#1792=CIRCLE('',#5801,5.5312722601991);
#1793=CIRCLE('',#5802,5.53127226019911);
#1794=CIRCLE('',#5803,0.405000000000004);
#1795=CIRCLE('',#5804,18.5625000000026);
#1796=CIRCLE('',#5805,5.53127226019917);
#1797=CIRCLE('',#5806,5.5312722601991);
#1798=CIRCLE('',#5807,0.405000000000001);
#1799=CIRCLE('',#5808,18.5625000000014);
#1800=CIRCLE('',#5809,5.53127226019908);
#1801=CIRCLE('',#5810,5.53127226019907);
#1802=CIRCLE('',#5811,0.405000000000004);
#1803=CIRCLE('',#5812,18.5624999999963);
#1804=CIRCLE('',#5813,5.53127226019908);
#1805=CIRCLE('',#5814,5.53127226019914);
#1806=CIRCLE('',#5815,0.405000000000001);
#1807=CIRCLE('',#5816,18.5625000000105);
#1808=CIRCLE('',#5817,5.53127226019909);
#1809=CIRCLE('',#5818,0.404999999999999);
#1810=CIRCLE('',#5819,18.5625000000053);
#1811=CIRCLE('',#5820,5.53127226019914);
#1812=CIRCLE('',#5821,0.405);
#1813=CIRCLE('',#5822,18.5624999999925);
#1814=CIRCLE('',#5823,0.405000000000001);
#1815=CIRCLE('',#5824,5.53127226019911);
#1816=CIRCLE('',#5825,5.53127226019916);
#1817=CIRCLE('',#5826,0.405000000000002);
#1818=CIRCLE('',#5827,18.5625000000065);
#1819=CIRCLE('',#5828,0.404999999999998);
#1820=CIRCLE('',#5829,5.53127226019912);
#1821=CIRCLE('',#5830,5.53127226019915);
#1822=CIRCLE('',#5831,0.404999999999998);
#1823=CIRCLE('',#5832,18.5625000000123);
#1824=CIRCLE('',#5833,0.405000000000006);
#1825=CIRCLE('',#5834,5.53127226019916);
#1826=CIRCLE('',#5835,5.53127226019912);
#1827=CIRCLE('',#5836,0.404999999999996);
#1828=CIRCLE('',#5837,18.5624999999983);
#1829=CIRCLE('',#5838,0.404999999999997);
#1830=CIRCLE('',#5839,5.53127226019917);
#1831=CIRCLE('',#5840,5.53127226019916);
#1832=CIRCLE('',#5841,0.405000000000008);
#1833=CIRCLE('',#5842,18.5625000000143);
#1834=CIRCLE('',#5843,0.404999999999994);
#1835=CIRCLE('',#5844,5.53127226019913);
#1836=CIRCLE('',#5845,5.53127226019921);
#1837=CIRCLE('',#5846,0.404999999999999);
#1838=CIRCLE('',#5847,18.5625000000044);
#1839=CIRCLE('',#5848,0.405000000000003);
#1840=CIRCLE('',#5849,5.5312722601991);
#1841=CIRCLE('',#5850,5.53127226019908);
#1842=CIRCLE('',#5851,0.404999999999999);
#1843=CIRCLE('',#5852,18.5625000000007);
#1844=CIRCLE('',#5853,0.405000000000003);
#1845=CIRCLE('',#5854,5.53127226019911);
#1846=CIRCLE('',#5855,5.53127226019911);
#1847=CIRCLE('',#5856,0.404999999999999);
#1848=CIRCLE('',#5857,18.5624999999966);
#1849=CIRCLE('',#5858,0.405000000000003);
#1850=CIRCLE('',#5859,5.53127226019913);
#1851=CIRCLE('',#5860,5.5312722601991);
#1852=CIRCLE('',#5861,0.405000000000002);
#1853=CIRCLE('',#5862,18.5625000000035);
#1854=CIRCLE('',#5863,0.404999999999999);
#1855=CIRCLE('',#5864,5.5312722601991);
#1856=CIRCLE('',#5865,5.53127226019911);
#1857=CIRCLE('',#5866,0.404999999999999);
#1858=CIRCLE('',#5867,18.562500000001);
#1859=CIRCLE('',#5868,0.405000000000003);
#1860=CIRCLE('',#5869,5.53127226019909);
#1861=CIRCLE('',#5870,5.53127226019911);
#1862=CIRCLE('',#5871,0.405000000000001);
#1863=CIRCLE('',#5872,18.562499999997);
#1864=CIRCLE('',#5873,0.405000000000003);
#1865=CIRCLE('',#5874,5.5312722601991);
#1866=CIRCLE('',#5875,5.53127226019909);
#1867=CIRCLE('',#5876,0.404999999999999);
#1868=CIRCLE('',#5877,18.5624999999987);
#1869=CIRCLE('',#5878,0.404999999999999);
#1967=VERTEX_POINT('',#8115);
#1968=VERTEX_POINT('',#8116);
#1969=VERTEX_POINT('',#8118);
#1970=VERTEX_POINT('',#8120);
#1971=VERTEX_POINT('',#8124);
#1972=VERTEX_POINT('',#8125);
#1973=VERTEX_POINT('',#8127);
#1974=VERTEX_POINT('',#8129);
#1975=VERTEX_POINT('',#8133);
#1976=VERTEX_POINT('',#8135);
#1977=VERTEX_POINT('',#8139);
#1978=VERTEX_POINT('',#8140);
#1979=VERTEX_POINT('',#8142);
#1980=VERTEX_POINT('',#8144);
#1981=VERTEX_POINT('',#8148);
#1982=VERTEX_POINT('',#8150);
#1983=VERTEX_POINT('',#8154);
#1984=VERTEX_POINT('',#8155);
#1985=VERTEX_POINT('',#8157);
#1986=VERTEX_POINT('',#8159);
#1987=VERTEX_POINT('',#8163);
#1988=VERTEX_POINT('',#8165);
#1989=VERTEX_POINT('',#8169);
#1990=VERTEX_POINT('',#8170);
#1991=VERTEX_POINT('',#8172);
#1992=VERTEX_POINT('',#8174);
#1993=VERTEX_POINT('',#8178);
#1994=VERTEX_POINT('',#8180);
#1995=VERTEX_POINT('',#8184);
#1996=VERTEX_POINT('',#8185);
#1997=VERTEX_POINT('',#8187);
#1998=VERTEX_POINT('',#8189);
#1999=VERTEX_POINT('',#8193);
#2000=VERTEX_POINT('',#8194);
#2001=VERTEX_POINT('',#8196);
#2002=VERTEX_POINT('',#8198);
#2003=VERTEX_POINT('',#8202);
#2004=VERTEX_POINT('',#8203);
#2005=VERTEX_POINT('',#8205);
#2006=VERTEX_POINT('',#8207);
#2007=VERTEX_POINT('',#8211);
#2008=VERTEX_POINT('',#8212);
#2009=VERTEX_POINT('',#8214);
#2010=VERTEX_POINT('',#8216);
#2011=VERTEX_POINT('',#8220);
#2012=VERTEX_POINT('',#8221);
#2013=VERTEX_POINT('',#8223);
#2014=VERTEX_POINT('',#8225);
#2015=VERTEX_POINT('',#8229);
#2016=VERTEX_POINT('',#8230);
#2017=VERTEX_POINT('',#8232);
#2018=VERTEX_POINT('',#8234);
#2019=VERTEX_POINT('',#8238);
#2020=VERTEX_POINT('',#8239);
#2021=VERTEX_POINT('',#8241);
#2022=VERTEX_POINT('',#8243);
#2023=VERTEX_POINT('',#8247);
#2024=VERTEX_POINT('',#8248);
#2025=VERTEX_POINT('',#8250);
#2026=VERTEX_POINT('',#8252);
#2027=VERTEX_POINT('',#8256);
#2028=VERTEX_POINT('',#8257);
#2029=VERTEX_POINT('',#8259);
#2030=VERTEX_POINT('',#8261);
#2031=VERTEX_POINT('',#8265);
#2032=VERTEX_POINT('',#8266);
#2033=VERTEX_POINT('',#8268);
#2034=VERTEX_POINT('',#8270);
#2035=VERTEX_POINT('',#8274);
#2036=VERTEX_POINT('',#8275);
#2037=VERTEX_POINT('',#8277);
#2038=VERTEX_POINT('',#8279);
#2039=VERTEX_POINT('',#8283);
#2040=VERTEX_POINT('',#8284);
#2041=VERTEX_POINT('',#8286);
#2042=VERTEX_POINT('',#8288);
#2043=VERTEX_POINT('',#8292);
#2044=VERTEX_POINT('',#8293);
#2045=VERTEX_POINT('',#8295);
#2046=VERTEX_POINT('',#8297);
#2047=VERTEX_POINT('',#8301);
#2048=VERTEX_POINT('',#8302);
#2049=VERTEX_POINT('',#8304);
#2050=VERTEX_POINT('',#8306);
#2051=VERTEX_POINT('',#8310);
#2052=VERTEX_POINT('',#8311);
#2053=VERTEX_POINT('',#8313);
#2054=VERTEX_POINT('',#8315);
#2055=VERTEX_POINT('',#8319);
#2056=VERTEX_POINT('',#8320);
#2057=VERTEX_POINT('',#8322);
#2058=VERTEX_POINT('',#8324);
#2059=VERTEX_POINT('',#8328);
#2060=VERTEX_POINT('',#8329);
#2061=VERTEX_POINT('',#8331);
#2062=VERTEX_POINT('',#8333);
#2063=VERTEX_POINT('',#8337);
#2064=VERTEX_POINT('',#8338);
#2065=VERTEX_POINT('',#8340);
#2066=VERTEX_POINT('',#8342);
#2067=VERTEX_POINT('',#8346);
#2068=VERTEX_POINT('',#8347);
#2069=VERTEX_POINT('',#8349);
#2070=VERTEX_POINT('',#8351);
#2071=VERTEX_POINT('',#8355);
#2072=VERTEX_POINT('',#8356);
#2073=VERTEX_POINT('',#8358);
#2074=VERTEX_POINT('',#8360);
#2075=VERTEX_POINT('',#8364);
#2076=VERTEX_POINT('',#8365);
#2077=VERTEX_POINT('',#8367);
#2078=VERTEX_POINT('',#8369);
#2079=VERTEX_POINT('',#8373);
#2080=VERTEX_POINT('',#8374);
#2081=VERTEX_POINT('',#8376);
#2082=VERTEX_POINT('',#8378);
#2083=VERTEX_POINT('',#8382);
#2084=VERTEX_POINT('',#8383);
#2085=VERTEX_POINT('',#8385);
#2086=VERTEX_POINT('',#8387);
#2087=VERTEX_POINT('',#8391);
#2088=VERTEX_POINT('',#8392);
#2089=VERTEX_POINT('',#8394);
#2090=VERTEX_POINT('',#8396);
#2091=VERTEX_POINT('',#8400);
#2092=VERTEX_POINT('',#8402);
#2093=VERTEX_POINT('',#8406);
#2094=VERTEX_POINT('',#8408);
#2095=VERTEX_POINT('',#8412);
#2096=VERTEX_POINT('',#8414);
#2097=VERTEX_POINT('',#8418);
#2098=VERTEX_POINT('',#8419);
#2099=VERTEX_POINT('',#8421);
#2100=VERTEX_POINT('',#8423);
#2101=VERTEX_POINT('',#8427);
#2102=VERTEX_POINT('',#8428);
#2103=VERTEX_POINT('',#8430);
#2104=VERTEX_POINT('',#8432);
#2105=VERTEX_POINT('',#8436);
#2106=VERTEX_POINT('',#8437);
#2107=VERTEX_POINT('',#8439);
#2108=VERTEX_POINT('',#8441);
#2109=VERTEX_POINT('',#8445);
#2110=VERTEX_POINT('',#8446);
#2111=VERTEX_POINT('',#8448);
#2112=VERTEX_POINT('',#8450);
#2113=VERTEX_POINT('',#8454);
#2114=VERTEX_POINT('',#8455);
#2115=VERTEX_POINT('',#8457);
#2116=VERTEX_POINT('',#8459);
#2117=VERTEX_POINT('',#8463);
#2118=VERTEX_POINT('',#8464);
#2119=VERTEX_POINT('',#8466);
#2120=VERTEX_POINT('',#8468);
#2121=VERTEX_POINT('',#8472);
#2122=VERTEX_POINT('',#8473);
#2123=VERTEX_POINT('',#8475);
#2124=VERTEX_POINT('',#8477);
#2125=VERTEX_POINT('',#8481);
#2126=VERTEX_POINT('',#8482);
#2127=VERTEX_POINT('',#8484);
#2128=VERTEX_POINT('',#8486);
#2129=VERTEX_POINT('',#8490);
#2130=VERTEX_POINT('',#8491);
#2131=VERTEX_POINT('',#8493);
#2132=VERTEX_POINT('',#8495);
#2133=VERTEX_POINT('',#8499);
#2134=VERTEX_POINT('',#8500);
#2135=VERTEX_POINT('',#8502);
#2136=VERTEX_POINT('',#8504);
#2137=VERTEX_POINT('',#8508);
#2138=VERTEX_POINT('',#8509);
#2139=VERTEX_POINT('',#8511);
#2140=VERTEX_POINT('',#8513);
#2141=VERTEX_POINT('',#8517);
#2142=VERTEX_POINT('',#8518);
#2143=VERTEX_POINT('',#8520);
#2144=VERTEX_POINT('',#8522);
#2145=VERTEX_POINT('',#8526);
#2146=VERTEX_POINT('',#8528);
#2147=VERTEX_POINT('',#8530);
#2148=VERTEX_POINT('',#8532);
#2149=VERTEX_POINT('',#8535);
#2150=VERTEX_POINT('',#8537);
#2151=VERTEX_POINT('',#8539);
#2152=VERTEX_POINT('',#8541);
#2153=VERTEX_POINT('',#8544);
#2154=VERTEX_POINT('',#8546);
#2155=VERTEX_POINT('',#8548);
#2156=VERTEX_POINT('',#8550);
#2157=VERTEX_POINT('',#8553);
#2158=VERTEX_POINT('',#8555);
#2159=VERTEX_POINT('',#8557);
#2160=VERTEX_POINT('',#8559);
#2161=VERTEX_POINT('',#8562);
#2162=VERTEX_POINT('',#8564);
#2163=VERTEX_POINT('',#8566);
#2164=VERTEX_POINT('',#8568);
#2165=VERTEX_POINT('',#8571);
#2166=VERTEX_POINT('',#8573);
#2167=VERTEX_POINT('',#8575);
#2168=VERTEX_POINT('',#8577);
#2169=VERTEX_POINT('',#8580);
#2170=VERTEX_POINT('',#8582);
#2171=VERTEX_POINT('',#8584);
#2172=VERTEX_POINT('',#8586);
#2173=VERTEX_POINT('',#8589);
#2174=VERTEX_POINT('',#8591);
#2175=VERTEX_POINT('',#8593);
#2176=VERTEX_POINT('',#8595);
#2177=VERTEX_POINT('',#8598);
#2178=VERTEX_POINT('',#8600);
#2179=VERTEX_POINT('',#8602);
#2180=VERTEX_POINT('',#8604);
#2181=VERTEX_POINT('',#8607);
#2182=VERTEX_POINT('',#8609);
#2183=VERTEX_POINT('',#8611);
#2184=VERTEX_POINT('',#8613);
#2185=VERTEX_POINT('',#8616);
#2186=VERTEX_POINT('',#8618);
#2187=VERTEX_POINT('',#8620);
#2188=VERTEX_POINT('',#8622);
#2189=VERTEX_POINT('',#8625);
#2190=VERTEX_POINT('',#8627);
#2191=VERTEX_POINT('',#8629);
#2192=VERTEX_POINT('',#8631);
#2193=VERTEX_POINT('',#8634);
#2194=VERTEX_POINT('',#8636);
#2195=VERTEX_POINT('',#8639);
#2196=VERTEX_POINT('',#8641);
#2197=VERTEX_POINT('',#8645);
#2198=VERTEX_POINT('',#8647);
#2199=VERTEX_POINT('',#8651);
#2200=VERTEX_POINT('',#8653);
#2201=VERTEX_POINT('',#8657);
#2202=VERTEX_POINT('',#8659);
#2203=VERTEX_POINT('',#8663);
#2204=VERTEX_POINT('',#8665);
#2205=VERTEX_POINT('',#8669);
#2206=VERTEX_POINT('',#8671);
#2207=VERTEX_POINT('',#8674);
#2208=VERTEX_POINT('',#8676);
#2209=VERTEX_POINT('',#8680);
#2210=VERTEX_POINT('',#8682);
#2211=VERTEX_POINT('',#8686);
#2212=VERTEX_POINT('',#8688);
#2213=VERTEX_POINT('',#8692);
#2214=VERTEX_POINT('',#8694);
#2215=VERTEX_POINT('',#8698);
#2216=VERTEX_POINT('',#8700);
#2217=VERTEX_POINT('',#8704);
#2218=VERTEX_POINT('',#8706);
#2219=VERTEX_POINT('',#8709);
#2220=VERTEX_POINT('',#8711);
#2221=VERTEX_POINT('',#8714);
#2222=VERTEX_POINT('',#8716);
#2223=VERTEX_POINT('',#8718);
#2224=VERTEX_POINT('',#8720);
#2225=VERTEX_POINT('',#8722);
#2226=VERTEX_POINT('',#8725);
#2227=VERTEX_POINT('',#8727);
#2228=VERTEX_POINT('',#8729);
#2229=VERTEX_POINT('',#8731);
#2230=VERTEX_POINT('',#8734);
#2231=VERTEX_POINT('',#8736);
#2232=VERTEX_POINT('',#8738);
#2233=VERTEX_POINT('',#8740);
#2234=VERTEX_POINT('',#8743);
#2235=VERTEX_POINT('',#8745);
#2236=VERTEX_POINT('',#8747);
#2237=VERTEX_POINT('',#8749);
#2238=VERTEX_POINT('',#8752);
#2239=VERTEX_POINT('',#8753);
#2240=VERTEX_POINT('',#8758);
#2241=VERTEX_POINT('',#8760);
#2242=VERTEX_POINT('',#8762);
#2243=VERTEX_POINT('',#8764);
#2244=VERTEX_POINT('',#8766);
#2245=VERTEX_POINT('',#8769);
#2246=VERTEX_POINT('',#8771);
#2247=VERTEX_POINT('',#8773);
#2248=VERTEX_POINT('',#8775);
#2249=VERTEX_POINT('',#8778);
#2250=VERTEX_POINT('',#8780);
#2251=VERTEX_POINT('',#8782);
#2252=VERTEX_POINT('',#8784);
#2253=VERTEX_POINT('',#8787);
#2254=VERTEX_POINT('',#8789);
#2255=VERTEX_POINT('',#8791);
#2256=VERTEX_POINT('',#8793);
#2257=VERTEX_POINT('',#8795);
#2258=VERTEX_POINT('',#8798);
#2259=VERTEX_POINT('',#8800);
#2260=VERTEX_POINT('',#8803);
#2261=VERTEX_POINT('',#8805);
#2262=VERTEX_POINT('',#8809);
#2263=VERTEX_POINT('',#8811);
#2264=VERTEX_POINT('',#8815);
#2265=VERTEX_POINT('',#8817);
#2266=VERTEX_POINT('',#8821);
#2267=VERTEX_POINT('',#8823);
#2268=VERTEX_POINT('',#8827);
#2269=VERTEX_POINT('',#8829);
#2270=VERTEX_POINT('',#8833);
#2271=VERTEX_POINT('',#8835);
#2272=VERTEX_POINT('',#8838);
#2273=VERTEX_POINT('',#8840);
#2274=VERTEX_POINT('',#8844);
#2275=VERTEX_POINT('',#8846);
#2276=VERTEX_POINT('',#8850);
#2277=VERTEX_POINT('',#8852);
#2278=VERTEX_POINT('',#8856);
#2279=VERTEX_POINT('',#8858);
#2280=VERTEX_POINT('',#8862);
#2281=VERTEX_POINT('',#8864);
#2282=VERTEX_POINT('',#8868);
#2283=VERTEX_POINT('',#8870);
#2284=VERTEX_POINT('',#8873);
#2285=VERTEX_POINT('',#8875);
#2286=VERTEX_POINT('',#8878);
#2287=VERTEX_POINT('',#8880);
#2288=VERTEX_POINT('',#8882);
#2289=VERTEX_POINT('',#8884);
#2290=VERTEX_POINT('',#8887);
#2291=VERTEX_POINT('',#8889);
#2292=VERTEX_POINT('',#8891);
#2293=VERTEX_POINT('',#8893);
#2294=VERTEX_POINT('',#8896);
#2295=VERTEX_POINT('',#8898);
#2296=VERTEX_POINT('',#8900);
#2297=VERTEX_POINT('',#8902);
#2298=VERTEX_POINT('',#8905);
#2299=VERTEX_POINT('',#8907);
#2300=VERTEX_POINT('',#8909);
#2301=VERTEX_POINT('',#8911);
#2302=VERTEX_POINT('',#8914);
#2303=VERTEX_POINT('',#8916);
#2304=VERTEX_POINT('',#8918);
#2305=VERTEX_POINT('',#8920);
#2306=VERTEX_POINT('',#8923);
#2307=VERTEX_POINT('',#8925);
#2308=VERTEX_POINT('',#8927);
#2309=VERTEX_POINT('',#8929);
#2310=VERTEX_POINT('',#8932);
#2311=VERTEX_POINT('',#8934);
#2312=VERTEX_POINT('',#8936);
#2313=VERTEX_POINT('',#8938);
#2314=VERTEX_POINT('',#8941);
#2315=VERTEX_POINT('',#8943);
#2316=VERTEX_POINT('',#8945);
#2317=VERTEX_POINT('',#8947);
#2318=VERTEX_POINT('',#8950);
#2319=VERTEX_POINT('',#8952);
#2320=VERTEX_POINT('',#8954);
#2321=VERTEX_POINT('',#8956);
#2322=VERTEX_POINT('',#8959);
#2323=VERTEX_POINT('',#8961);
#2324=VERTEX_POINT('',#8963);
#2325=VERTEX_POINT('',#8965);
#2326=VERTEX_POINT('',#8968);
#2327=VERTEX_POINT('',#8970);
#2328=VERTEX_POINT('',#8972);
#2329=VERTEX_POINT('',#8974);
#2330=VERTEX_POINT('',#8977);
#2331=VERTEX_POINT('',#8979);
#2332=VERTEX_POINT('',#8981);
#2333=VERTEX_POINT('',#8984);
#2334=VERTEX_POINT('',#8986);
#2512=EDGE_CURVE('',#1967,#1968,#1508,.T.);
#2513=EDGE_CURVE('',#1967,#1969,#938,.T.);
#2514=EDGE_CURVE('',#1969,#1970,#1509,.T.);
#2515=EDGE_CURVE('',#1970,#1968,#939,.T.);
#2516=EDGE_CURVE('',#1971,#1972,#1510,.T.);
#2517=EDGE_CURVE('',#1973,#1971,#940,.T.);
#2518=EDGE_CURVE('',#1974,#1973,#1511,.T.);
#2519=EDGE_CURVE('',#1972,#1974,#941,.T.);
#2520=EDGE_CURVE('',#1975,#1974,#1512,.T.);
#2521=EDGE_CURVE('',#1976,#1975,#942,.T.);
#2522=EDGE_CURVE('',#1976,#1972,#1513,.T.);
#2523=EDGE_CURVE('',#1977,#1978,#1514,.T.);
#2524=EDGE_CURVE('',#1979,#1977,#943,.T.);
#2525=EDGE_CURVE('',#1980,#1979,#1515,.T.);
#2526=EDGE_CURVE('',#1978,#1980,#944,.T.);
#2527=EDGE_CURVE('',#1981,#1980,#1516,.T.);
#2528=EDGE_CURVE('',#1982,#1981,#945,.T.);
#2529=EDGE_CURVE('',#1982,#1978,#1517,.T.);
#2530=EDGE_CURVE('',#1983,#1984,#1518,.T.);
#2531=EDGE_CURVE('',#1985,#1983,#946,.T.);
#2532=EDGE_CURVE('',#1986,#1985,#1519,.T.);
#2533=EDGE_CURVE('',#1984,#1986,#947,.T.);
#2534=EDGE_CURVE('',#1985,#1987,#1520,.T.);
#2535=EDGE_CURVE('',#1983,#1988,#1521,.T.);
#2536=EDGE_CURVE('',#1987,#1988,#948,.T.);
#2537=EDGE_CURVE('',#1989,#1990,#1522,.T.);
#2538=EDGE_CURVE('',#1991,#1989,#949,.T.);
#2539=EDGE_CURVE('',#1992,#1991,#1523,.T.);
#2540=EDGE_CURVE('',#1990,#1992,#950,.T.);
#2541=EDGE_CURVE('',#1991,#1993,#1524,.T.);
#2542=EDGE_CURVE('',#1989,#1994,#1525,.T.);
#2543=EDGE_CURVE('',#1993,#1994,#951,.T.);
#2544=EDGE_CURVE('',#1995,#1996,#1526,.T.);
#2545=EDGE_CURVE('',#1997,#1995,#952,.T.);
#2546=EDGE_CURVE('',#1998,#1997,#1527,.T.);
#2547=EDGE_CURVE('',#1996,#1998,#953,.T.);
#2548=EDGE_CURVE('',#1999,#2000,#1528,.T.);
#2549=EDGE_CURVE('',#2001,#1999,#954,.T.);
#2550=EDGE_CURVE('',#2002,#2001,#1529,.T.);
#2551=EDGE_CURVE('',#2000,#2002,#955,.T.);
#2552=EDGE_CURVE('',#2003,#2004,#1530,.T.);
#2553=EDGE_CURVE('',#2005,#2003,#956,.T.);
#2554=EDGE_CURVE('',#2006,#2005,#1531,.T.);
#2555=EDGE_CURVE('',#2004,#2006,#957,.T.);
#2556=EDGE_CURVE('',#2007,#2008,#1532,.T.);
#2557=EDGE_CURVE('',#2009,#2007,#958,.T.);
#2558=EDGE_CURVE('',#2010,#2009,#1533,.T.);
#2559=EDGE_CURVE('',#2008,#2010,#959,.T.);
#2560=EDGE_CURVE('',#2011,#2012,#1534,.T.);
#2561=EDGE_CURVE('',#2013,#2011,#960,.T.);
#2562=EDGE_CURVE('',#2014,#2013,#1535,.T.);
#2563=EDGE_CURVE('',#2012,#2014,#961,.T.);
#2564=EDGE_CURVE('',#2015,#2016,#1536,.T.);
#2565=EDGE_CURVE('',#2017,#2015,#962,.T.);
#2566=EDGE_CURVE('',#2018,#2017,#1537,.T.);
#2567=EDGE_CURVE('',#2016,#2018,#963,.T.);
#2568=EDGE_CURVE('',#2019,#2020,#1538,.T.);
#2569=EDGE_CURVE('',#2021,#2019,#964,.T.);
#2570=EDGE_CURVE('',#2022,#2021,#1539,.T.);
#2571=EDGE_CURVE('',#2020,#2022,#965,.T.);
#2572=EDGE_CURVE('',#2023,#2024,#1540,.T.);
#2573=EDGE_CURVE('',#2025,#2023,#966,.T.);
#2574=EDGE_CURVE('',#2026,#2025,#1541,.T.);
#2575=EDGE_CURVE('',#2024,#2026,#967,.T.);
#2576=EDGE_CURVE('',#2027,#2028,#1542,.T.);
#2577=EDGE_CURVE('',#2029,#2027,#968,.T.);
#2578=EDGE_CURVE('',#2030,#2029,#1543,.T.);
#2579=EDGE_CURVE('',#2028,#2030,#969,.T.);
#2580=EDGE_CURVE('',#2031,#2032,#1544,.T.);
#2581=EDGE_CURVE('',#2033,#2031,#970,.T.);
#2582=EDGE_CURVE('',#2034,#2033,#1545,.T.);
#2583=EDGE_CURVE('',#2032,#2034,#971,.T.);
#2584=EDGE_CURVE('',#2035,#2036,#1546,.T.);
#2585=EDGE_CURVE('',#2035,#2037,#972,.T.);
#2586=EDGE_CURVE('',#2037,#2038,#1547,.T.);
#2587=EDGE_CURVE('',#2038,#2036,#973,.T.);
#2588=EDGE_CURVE('',#2039,#2040,#1548,.T.);
#2589=EDGE_CURVE('',#2039,#2041,#974,.T.);
#2590=EDGE_CURVE('',#2041,#2042,#1549,.T.);
#2591=EDGE_CURVE('',#2042,#2040,#975,.T.);
#2592=EDGE_CURVE('',#2043,#2044,#1550,.T.);
#2593=EDGE_CURVE('',#2044,#2045,#976,.T.);
#2594=EDGE_CURVE('',#2046,#2045,#1551,.T.);
#2595=EDGE_CURVE('',#2046,#2043,#977,.T.);
#2596=EDGE_CURVE('',#2047,#2048,#1552,.T.);
#2597=EDGE_CURVE('',#2047,#2049,#978,.T.);
#2598=EDGE_CURVE('',#2049,#2050,#1553,.T.);
#2599=EDGE_CURVE('',#2050,#2048,#979,.T.);
#2600=EDGE_CURVE('',#2051,#2052,#1554,.T.);
#2601=EDGE_CURVE('',#2051,#2053,#980,.T.);
#2602=EDGE_CURVE('',#2053,#2054,#1555,.T.);
#2603=EDGE_CURVE('',#2054,#2052,#981,.T.);
#2604=EDGE_CURVE('',#2055,#2056,#1556,.T.);
#2605=EDGE_CURVE('',#2056,#2057,#982,.T.);
#2606=EDGE_CURVE('',#2058,#2057,#1557,.T.);
#2607=EDGE_CURVE('',#2058,#2055,#983,.T.);
#2608=EDGE_CURVE('',#2059,#2060,#1558,.T.);
#2609=EDGE_CURVE('',#2060,#2061,#984,.T.);
#2610=EDGE_CURVE('',#2062,#2061,#1559,.T.);
#2611=EDGE_CURVE('',#2062,#2059,#985,.T.);
#2612=EDGE_CURVE('',#2063,#2064,#1560,.T.);
#2613=EDGE_CURVE('',#2064,#2065,#986,.T.);
#2614=EDGE_CURVE('',#2066,#2065,#1561,.T.);
#2615=EDGE_CURVE('',#2066,#2063,#987,.T.);
#2616=EDGE_CURVE('',#2067,#2068,#1562,.T.);
#2617=EDGE_CURVE('',#2067,#2069,#988,.T.);
#2618=EDGE_CURVE('',#2069,#2070,#1563,.T.);
#2619=EDGE_CURVE('',#2070,#2068,#989,.T.);
#2620=EDGE_CURVE('',#2071,#2072,#1564,.T.);
#2621=EDGE_CURVE('',#2071,#2073,#990,.T.);
#2622=EDGE_CURVE('',#2073,#2074,#1565,.T.);
#2623=EDGE_CURVE('',#2074,#2072,#991,.T.);
#2624=EDGE_CURVE('',#2075,#2076,#1566,.T.);
#2625=EDGE_CURVE('',#2076,#2077,#992,.T.);
#2626=EDGE_CURVE('',#2078,#2077,#1567,.T.);
#2627=EDGE_CURVE('',#2078,#2075,#993,.T.);
#2628=EDGE_CURVE('',#2079,#2080,#1568,.T.);
#2629=EDGE_CURVE('',#2080,#2081,#994,.T.);
#2630=EDGE_CURVE('',#2082,#2081,#1569,.T.);
#2631=EDGE_CURVE('',#2082,#2079,#995,.T.);
#2632=EDGE_CURVE('',#2083,#2084,#1570,.T.);
#2633=EDGE_CURVE('',#2084,#2085,#996,.T.);
#2634=EDGE_CURVE('',#2086,#2085,#1571,.T.);
#2635=EDGE_CURVE('',#2086,#2083,#997,.T.);
#2636=EDGE_CURVE('',#2087,#2088,#1572,.T.);
#2637=EDGE_CURVE('',#2088,#2089,#998,.T.);
#2638=EDGE_CURVE('',#2090,#2089,#1573,.T.);
#2639=EDGE_CURVE('',#2090,#2087,#999,.T.);
#2640=EDGE_CURVE('',#1975,#2091,#1574,.T.);
#2641=EDGE_CURVE('',#2091,#2092,#1000,.T.);
#2642=EDGE_CURVE('',#1976,#2092,#1575,.T.);
#2643=EDGE_CURVE('',#1981,#2093,#1576,.T.);
#2644=EDGE_CURVE('',#2093,#2094,#1001,.T.);
#2645=EDGE_CURVE('',#1982,#2094,#1577,.T.);
#2646=EDGE_CURVE('',#2095,#1994,#1578,.T.);
#2647=EDGE_CURVE('',#2095,#2096,#1002,.T.);
#2648=EDGE_CURVE('',#2096,#1993,#1579,.T.);
#2649=EDGE_CURVE('',#2097,#2098,#1580,.T.);
#2650=EDGE_CURVE('',#2097,#2099,#1003,.T.);
#2651=EDGE_CURVE('',#2099,#2100,#1581,.T.);
#2652=EDGE_CURVE('',#2100,#2098,#1004,.T.);
#2653=EDGE_CURVE('',#2101,#2102,#1582,.T.);
#2654=EDGE_CURVE('',#2101,#2103,#1005,.T.);
#2655=EDGE_CURVE('',#2103,#2104,#1583,.T.);
#2656=EDGE_CURVE('',#2104,#2102,#1006,.T.);
#2657=EDGE_CURVE('',#2105,#2106,#1584,.T.);
#2658=EDGE_CURVE('',#2106,#2107,#1007,.T.);
#2659=EDGE_CURVE('',#2108,#2107,#1585,.T.);
#2660=EDGE_CURVE('',#2108,#2105,#1008,.T.);
#2661=EDGE_CURVE('',#2109,#2110,#1586,.T.);
#2662=EDGE_CURVE('',#2109,#2111,#1009,.T.);
#2663=EDGE_CURVE('',#2111,#2112,#1587,.T.);
#2664=EDGE_CURVE('',#2112,#2110,#1010,.T.);
#2665=EDGE_CURVE('',#2113,#2114,#1588,.T.);
#2666=EDGE_CURVE('',#2113,#2115,#1011,.T.);
#2667=EDGE_CURVE('',#2115,#2116,#1589,.T.);
#2668=EDGE_CURVE('',#2116,#2114,#1012,.T.);
#2669=EDGE_CURVE('',#2117,#2118,#1590,.T.);
#2670=EDGE_CURVE('',#2117,#2119,#1013,.T.);
#2671=EDGE_CURVE('',#2119,#2120,#1591,.T.);
#2672=EDGE_CURVE('',#2120,#2118,#1014,.T.);
#2673=EDGE_CURVE('',#2121,#2122,#1592,.T.);
#2674=EDGE_CURVE('',#2121,#2123,#1015,.T.);
#2675=EDGE_CURVE('',#2123,#2124,#1593,.T.);
#2676=EDGE_CURVE('',#2124,#2122,#1016,.T.);
#2677=EDGE_CURVE('',#2125,#2126,#1594,.T.);
#2678=EDGE_CURVE('',#2125,#2127,#1017,.T.);
#2679=EDGE_CURVE('',#2127,#2128,#1595,.T.);
#2680=EDGE_CURVE('',#2128,#2126,#1018,.T.);
#2681=EDGE_CURVE('',#2129,#2130,#1596,.T.);
#2682=EDGE_CURVE('',#2130,#2131,#1019,.T.);
#2683=EDGE_CURVE('',#2132,#2131,#1597,.T.);
#2684=EDGE_CURVE('',#2132,#2129,#1020,.T.);
#2685=EDGE_CURVE('',#2133,#2134,#1598,.T.);
#2686=EDGE_CURVE('',#2134,#2135,#1021,.T.);
#2687=EDGE_CURVE('',#2136,#2135,#1599,.T.);
#2688=EDGE_CURVE('',#2136,#2133,#1022,.T.);
#2689=EDGE_CURVE('',#2137,#2138,#1600,.T.);
#2690=EDGE_CURVE('',#2138,#2139,#1023,.T.);
#2691=EDGE_CURVE('',#2140,#2139,#1601,.T.);
#2692=EDGE_CURVE('',#2140,#2137,#1024,.T.);
#2693=EDGE_CURVE('',#2141,#2142,#1602,.T.);
#2694=EDGE_CURVE('',#2141,#2143,#1025,.T.);
#2695=EDGE_CURVE('',#2143,#2144,#1603,.T.);
#2696=EDGE_CURVE('',#2144,#2142,#1026,.T.);
#2697=EDGE_CURVE('',#2041,#2145,#1604,.T.);
#2698=EDGE_CURVE('',#2145,#2146,#1605,.T.);
#2699=EDGE_CURVE('',#2146,#2147,#1606,.T.);
#2700=EDGE_CURVE('',#2147,#2148,#1607,.T.);
#2701=EDGE_CURVE('',#2148,#2044,#1608,.T.);
#2702=EDGE_CURVE('',#2043,#2149,#1609,.T.);
#2703=EDGE_CURVE('',#2149,#2150,#1610,.T.);
#2704=EDGE_CURVE('',#2150,#2151,#1611,.T.);
#2705=EDGE_CURVE('',#2151,#2152,#1612,.T.);
#2706=EDGE_CURVE('',#2152,#2056,#1613,.T.);
#2707=EDGE_CURVE('',#2055,#2153,#1614,.T.);
#2708=EDGE_CURVE('',#2153,#2154,#1615,.T.);
#2709=EDGE_CURVE('',#2154,#2155,#1616,.T.);
#2710=EDGE_CURVE('',#2155,#2156,#1617,.T.);
#2711=EDGE_CURVE('',#2156,#2060,#1618,.T.);
#2712=EDGE_CURVE('',#2059,#2157,#1619,.T.);
#2713=EDGE_CURVE('',#2157,#2158,#1620,.T.);
#2714=EDGE_CURVE('',#2158,#2159,#1621,.T.);
#2715=EDGE_CURVE('',#2159,#2160,#1622,.T.);
#2716=EDGE_CURVE('',#2160,#2038,#1623,.T.);
#2717=EDGE_CURVE('',#2037,#2161,#1624,.T.);
#2718=EDGE_CURVE('',#2161,#2162,#1625,.T.);
#2719=EDGE_CURVE('',#2162,#2163,#1626,.T.);
#2720=EDGE_CURVE('',#2163,#2164,#1627,.T.);
#2721=EDGE_CURVE('',#2164,#2064,#1628,.T.);
#2722=EDGE_CURVE('',#2063,#2165,#1629,.T.);
#2723=EDGE_CURVE('',#2165,#2166,#1630,.T.);
#2724=EDGE_CURVE('',#2166,#2167,#1631,.T.);
#2725=EDGE_CURVE('',#2167,#2168,#1632,.T.);
#2726=EDGE_CURVE('',#2168,#2076,#1633,.T.);
#2727=EDGE_CURVE('',#2075,#2169,#1634,.T.);
#2728=EDGE_CURVE('',#2169,#2170,#1635,.T.);
#2729=EDGE_CURVE('',#2170,#2171,#1636,.T.);
#2730=EDGE_CURVE('',#2171,#2172,#1637,.T.);
#2731=EDGE_CURVE('',#2172,#2080,#1638,.T.);
#2732=EDGE_CURVE('',#2079,#2173,#1639,.T.);
#2733=EDGE_CURVE('',#2173,#2174,#1640,.T.);
#2734=EDGE_CURVE('',#2174,#2175,#1641,.T.);
#2735=EDGE_CURVE('',#2175,#2176,#1642,.T.);
#2736=EDGE_CURVE('',#2176,#2074,#1643,.T.);
#2737=EDGE_CURVE('',#2073,#2177,#1644,.T.);
#2738=EDGE_CURVE('',#2177,#2178,#1645,.T.);
#2739=EDGE_CURVE('',#2178,#2179,#1646,.T.);
#2740=EDGE_CURVE('',#2179,#2180,#1647,.T.);
#2741=EDGE_CURVE('',#2180,#2070,#1648,.T.);
#2742=EDGE_CURVE('',#2069,#2181,#1649,.T.);
#2743=EDGE_CURVE('',#2181,#2182,#1650,.T.);
#2744=EDGE_CURVE('',#2182,#2183,#1651,.T.);
#2745=EDGE_CURVE('',#2183,#2184,#1652,.T.);
#2746=EDGE_CURVE('',#2184,#2084,#1653,.T.);
#2747=EDGE_CURVE('',#2083,#2185,#1654,.T.);
#2748=EDGE_CURVE('',#2185,#2186,#1655,.T.);
#2749=EDGE_CURVE('',#2186,#2187,#1656,.T.);
#2750=EDGE_CURVE('',#2187,#2188,#1657,.T.);
#2751=EDGE_CURVE('',#2188,#2088,#1658,.T.);
#2752=EDGE_CURVE('',#2087,#2189,#1659,.T.);
#2753=EDGE_CURVE('',#2189,#2190,#1660,.T.);
#2754=EDGE_CURVE('',#2190,#2191,#1661,.T.);
#2755=EDGE_CURVE('',#2191,#2192,#1662,.T.);
#2756=EDGE_CURVE('',#2192,#2091,#1663,.T.);
#2757=EDGE_CURVE('',#1973,#2193,#1664,.T.);
#2758=EDGE_CURVE('',#2193,#2194,#1665,.T.);
#2759=EDGE_CURVE('',#2194,#2093,#1666,.T.);
#2760=EDGE_CURVE('',#1979,#2195,#1667,.T.);
#2761=EDGE_CURVE('',#2195,#2196,#1668,.T.);
#2762=EDGE_CURVE('',#2196,#2130,#1669,.T.);
#2763=EDGE_CURVE('',#2129,#2026,#1670,.T.);
#2764=EDGE_CURVE('',#2025,#2197,#1671,.T.);
#2765=EDGE_CURVE('',#2197,#2198,#1672,.T.);
#2766=EDGE_CURVE('',#2198,#2128,#1673,.T.);
#2767=EDGE_CURVE('',#2127,#2022,#1674,.T.);
#2768=EDGE_CURVE('',#2021,#2199,#1675,.T.);
#2769=EDGE_CURVE('',#2199,#2200,#1676,.T.);
#2770=EDGE_CURVE('',#2200,#2134,#1677,.T.);
#2771=EDGE_CURVE('',#2133,#2030,#1678,.T.);
#2772=EDGE_CURVE('',#2029,#2201,#1679,.T.);
#2773=EDGE_CURVE('',#2201,#2202,#1680,.T.);
#2774=EDGE_CURVE('',#2202,#2138,#1681,.T.);
#2775=EDGE_CURVE('',#2137,#2034,#1682,.T.);
#2776=EDGE_CURVE('',#2033,#2203,#1683,.T.);
#2777=EDGE_CURVE('',#2203,#2204,#1684,.T.);
#2778=EDGE_CURVE('',#2204,#2124,#1685,.T.);
#2779=EDGE_CURVE('',#2123,#2018,#1686,.T.);
#2780=EDGE_CURVE('',#2017,#2205,#1687,.T.);
#2781=EDGE_CURVE('',#2205,#2206,#1688,.T.);
#2782=EDGE_CURVE('',#2206,#2120,#1689,.T.);
#2783=EDGE_CURVE('',#2119,#2207,#1690,.T.);
#2784=EDGE_CURVE('',#2207,#2208,#1691,.T.);
#2785=EDGE_CURVE('',#2208,#2014,#1692,.T.);
#2786=EDGE_CURVE('',#2013,#2116,#1693,.T.);
#2787=EDGE_CURVE('',#2115,#2209,#1694,.T.);
#2788=EDGE_CURVE('',#2209,#2210,#1695,.T.);
#2789=EDGE_CURVE('',#2210,#2010,#1696,.T.);
#2790=EDGE_CURVE('',#2009,#2112,#1697,.T.);
#2791=EDGE_CURVE('',#2111,#2211,#1698,.T.);
#2792=EDGE_CURVE('',#2211,#2212,#1699,.T.);
#2793=EDGE_CURVE('',#2212,#2006,#1700,.T.);
#2794=EDGE_CURVE('',#2005,#2104,#1701,.T.);
#2795=EDGE_CURVE('',#2103,#2213,#1702,.T.);
#2796=EDGE_CURVE('',#2213,#2214,#1703,.T.);
#2797=EDGE_CURVE('',#2214,#1998,#1704,.T.);
#2798=EDGE_CURVE('',#1997,#2106,#1705,.T.);
#2799=EDGE_CURVE('',#2105,#2215,#1706,.T.);
#2800=EDGE_CURVE('',#2215,#2216,#1707,.T.);
#2801=EDGE_CURVE('',#2216,#2002,#1708,.T.);
#2802=EDGE_CURVE('',#2001,#2100,#1709,.T.);
#2803=EDGE_CURVE('',#2099,#2217,#1710,.T.);
#2804=EDGE_CURVE('',#2217,#2218,#1711,.T.);
#2805=EDGE_CURVE('',#2218,#1992,#1712,.T.);
#2806=EDGE_CURVE('',#2096,#2219,#1713,.T.);
#2807=EDGE_CURVE('',#2219,#2220,#1714,.T.);
#2808=EDGE_CURVE('',#2220,#1986,#1715,.T.);
#2809=EDGE_CURVE('',#2221,#1987,#1716,.T.);
#2810=EDGE_CURVE('',#2221,#2222,#1717,.T.);
#2811=EDGE_CURVE('',#2222,#2223,#1718,.T.);
#2812=EDGE_CURVE('',#2223,#2224,#1719,.T.);
#2813=EDGE_CURVE('',#2224,#2225,#1720,.T.);
#2814=EDGE_CURVE('',#2225,#2144,#1721,.T.);
#2815=EDGE_CURVE('',#2143,#2226,#1722,.T.);
#2816=EDGE_CURVE('',#2226,#2227,#1723,.T.);
#2817=EDGE_CURVE('',#2227,#2228,#1724,.T.);
#2818=EDGE_CURVE('',#2228,#2229,#1725,.T.);
#2819=EDGE_CURVE('',#2229,#2054,#1726,.T.);
#2820=EDGE_CURVE('',#2053,#2230,#1727,.T.);
#2821=EDGE_CURVE('',#2230,#2231,#1728,.T.);
#2822=EDGE_CURVE('',#2231,#2232,#1729,.T.);
#2823=EDGE_CURVE('',#2232,#2233,#1730,.T.);
#2824=EDGE_CURVE('',#2233,#2050,#1731,.T.);
#2825=EDGE_CURVE('',#2049,#2234,#1732,.T.);
#2826=EDGE_CURVE('',#2234,#2235,#1733,.T.);
#2827=EDGE_CURVE('',#2235,#2236,#1734,.T.);
#2828=EDGE_CURVE('',#2236,#2237,#1735,.T.);
#2829=EDGE_CURVE('',#2237,#2042,#1736,.T.);
#2830=EDGE_CURVE('',#2238,#2239,#1027,.T.);
#2831=EDGE_CURVE('',#2239,#1967,#1028,.T.);
#2832=EDGE_CURVE('',#1968,#2238,#1029,.T.);
#2833=EDGE_CURVE('',#2039,#2240,#1737,.T.);
#2834=EDGE_CURVE('',#2241,#2040,#1738,.T.);
#2835=EDGE_CURVE('',#2241,#2242,#1739,.T.);
#2836=EDGE_CURVE('',#2243,#2242,#1740,.T.);
#2837=EDGE_CURVE('',#2243,#2244,#1741,.T.);
#2838=EDGE_CURVE('',#2047,#2244,#1742,.T.);
#2839=EDGE_CURVE('',#2245,#2048,#1743,.T.);
#2840=EDGE_CURVE('',#2245,#2246,#1744,.T.);
#2841=EDGE_CURVE('',#2247,#2246,#1745,.T.);
#2842=EDGE_CURVE('',#2247,#2248,#1746,.T.);
#2843=EDGE_CURVE('',#2051,#2248,#1747,.T.);
#2844=EDGE_CURVE('',#2249,#2052,#1748,.T.);
#2845=EDGE_CURVE('',#2249,#2250,#1749,.T.);
#2846=EDGE_CURVE('',#2251,#2250,#1750,.T.);
#2847=EDGE_CURVE('',#2251,#2252,#1751,.T.);
#2848=EDGE_CURVE('',#2141,#2252,#1752,.T.);
#2849=EDGE_CURVE('',#2253,#2142,#1753,.T.);
#2850=EDGE_CURVE('',#2253,#2254,#1754,.T.);
#2851=EDGE_CURVE('',#2255,#2254,#1755,.T.);
#2852=EDGE_CURVE('',#2255,#2256,#1756,.T.);
#2853=EDGE_CURVE('',#2257,#2256,#1757,.T.);
#2854=EDGE_CURVE('',#2257,#1988,#1758,.T.);
#2855=EDGE_CURVE('',#2258,#1984,#1759,.T.);
#2856=EDGE_CURVE('',#2258,#2259,#1760,.T.);
#2857=EDGE_CURVE('',#2095,#2259,#1761,.T.);
#2858=EDGE_CURVE('',#2260,#1990,#1762,.T.);
#2859=EDGE_CURVE('',#2260,#2261,#1763,.T.);
#2860=EDGE_CURVE('',#2097,#2261,#1764,.T.);
#2861=EDGE_CURVE('',#1999,#2098,#1765,.T.);
#2862=EDGE_CURVE('',#2262,#2000,#1766,.T.);
#2863=EDGE_CURVE('',#2262,#2263,#1767,.T.);
#2864=EDGE_CURVE('',#2108,#2263,#1768,.T.);
#2865=EDGE_CURVE('',#1995,#2107,#1769,.T.);
#2866=EDGE_CURVE('',#2264,#1996,#1770,.T.);
#2867=EDGE_CURVE('',#2264,#2265,#1771,.T.);
#2868=EDGE_CURVE('',#2101,#2265,#1772,.T.);
#2869=EDGE_CURVE('',#2003,#2102,#1773,.T.);
#2870=EDGE_CURVE('',#2266,#2004,#1774,.T.);
#2871=EDGE_CURVE('',#2266,#2267,#1775,.T.);
#2872=EDGE_CURVE('',#2109,#2267,#1776,.T.);
#2873=EDGE_CURVE('',#2007,#2110,#1777,.T.);
#2874=EDGE_CURVE('',#2268,#2008,#1778,.T.);
#2875=EDGE_CURVE('',#2268,#2269,#1779,.T.);
#2876=EDGE_CURVE('',#2113,#2269,#1780,.T.);
#2877=EDGE_CURVE('',#2011,#2114,#1781,.T.);
#2878=EDGE_CURVE('',#2270,#2012,#1782,.T.);
#2879=EDGE_CURVE('',#2270,#2271,#1783,.T.);
#2880=EDGE_CURVE('',#2117,#2271,#1784,.T.);
#2881=EDGE_CURVE('',#2272,#2118,#1785,.T.);
#2882=EDGE_CURVE('',#2272,#2273,#1786,.T.);
#2883=EDGE_CURVE('',#2015,#2273,#1787,.T.);
#2884=EDGE_CURVE('',#2121,#2016,#1788,.T.);
#2885=EDGE_CURVE('',#2274,#2122,#1789,.T.);
#2886=EDGE_CURVE('',#2274,#2275,#1790,.T.);
#2887=EDGE_CURVE('',#2031,#2275,#1791,.T.);
#2888=EDGE_CURVE('',#2140,#2032,#1792,.T.);
#2889=EDGE_CURVE('',#2276,#2139,#1793,.T.);
#2890=EDGE_CURVE('',#2276,#2277,#1794,.T.);
#2891=EDGE_CURVE('',#2027,#2277,#1795,.T.);
#2892=EDGE_CURVE('',#2136,#2028,#1796,.T.);
#2893=EDGE_CURVE('',#2278,#2135,#1797,.T.);
#2894=EDGE_CURVE('',#2278,#2279,#1798,.T.);
#2895=EDGE_CURVE('',#2019,#2279,#1799,.T.);
#2896=EDGE_CURVE('',#2125,#2020,#1800,.T.);
#2897=EDGE_CURVE('',#2280,#2126,#1801,.T.);
#2898=EDGE_CURVE('',#2280,#2281,#1802,.T.);
#2899=EDGE_CURVE('',#2023,#2281,#1803,.T.);
#2900=EDGE_CURVE('',#2132,#2024,#1804,.T.);
#2901=EDGE_CURVE('',#2282,#2131,#1805,.T.);
#2902=EDGE_CURVE('',#2282,#2283,#1806,.T.);
#2903=EDGE_CURVE('',#1977,#2283,#1807,.T.);
#2904=EDGE_CURVE('',#2284,#2094,#1808,.T.);
#2905=EDGE_CURVE('',#2284,#2285,#1809,.T.);
#2906=EDGE_CURVE('',#1971,#2285,#1810,.T.);
#2907=EDGE_CURVE('',#2286,#2092,#1811,.T.);
#2908=EDGE_CURVE('',#2286,#2287,#1812,.T.);
#2909=EDGE_CURVE('',#2288,#2287,#1813,.T.);
#2910=EDGE_CURVE('',#2288,#2289,#1814,.T.);
#2911=EDGE_CURVE('',#2090,#2289,#1815,.T.);
#2912=EDGE_CURVE('',#2290,#2089,#1816,.T.);
#2913=EDGE_CURVE('',#2290,#2291,#1817,.T.);
#2914=EDGE_CURVE('',#2292,#2291,#1818,.T.);
#2915=EDGE_CURVE('',#2292,#2293,#1819,.T.);
#2916=EDGE_CURVE('',#2086,#2293,#1820,.T.);
#2917=EDGE_CURVE('',#2294,#2085,#1821,.T.);
#2918=EDGE_CURVE('',#2294,#2295,#1822,.T.);
#2919=EDGE_CURVE('',#2296,#2295,#1823,.T.);
#2920=EDGE_CURVE('',#2296,#2297,#1824,.T.);
#2921=EDGE_CURVE('',#2067,#2297,#1825,.T.);
#2922=EDGE_CURVE('',#2298,#2068,#1826,.T.);
#2923=EDGE_CURVE('',#2298,#2299,#1827,.T.);
#2924=EDGE_CURVE('',#2300,#2299,#1828,.T.);
#2925=EDGE_CURVE('',#2300,#2301,#1829,.T.);
#2926=EDGE_CURVE('',#2071,#2301,#1830,.T.);
#2927=EDGE_CURVE('',#2302,#2072,#1831,.T.);
#2928=EDGE_CURVE('',#2302,#2303,#1832,.T.);
#2929=EDGE_CURVE('',#2304,#2303,#1833,.T.);
#2930=EDGE_CURVE('',#2304,#2305,#1834,.T.);
#2931=EDGE_CURVE('',#2082,#2305,#1835,.T.);
#2932=EDGE_CURVE('',#2306,#2081,#1836,.T.);
#2933=EDGE_CURVE('',#2306,#2307,#1837,.T.);
#2934=EDGE_CURVE('',#2308,#2307,#1838,.T.);
#2935=EDGE_CURVE('',#2308,#2309,#1839,.T.);
#2936=EDGE_CURVE('',#2078,#2309,#1840,.T.);
#2937=EDGE_CURVE('',#2310,#2077,#1841,.T.);
#2938=EDGE_CURVE('',#2310,#2311,#1842,.T.);
#2939=EDGE_CURVE('',#2312,#2311,#1843,.T.);
#2940=EDGE_CURVE('',#2312,#2313,#1844,.T.);
#2941=EDGE_CURVE('',#2066,#2313,#1845,.T.);
#2942=EDGE_CURVE('',#2314,#2065,#1846,.T.);
#2943=EDGE_CURVE('',#2314,#2315,#1847,.T.);
#2944=EDGE_CURVE('',#2316,#2315,#1848,.T.);
#2945=EDGE_CURVE('',#2316,#2317,#1849,.T.);
#2946=EDGE_CURVE('',#2035,#2317,#1850,.T.);
#2947=EDGE_CURVE('',#2318,#2036,#1851,.T.);
#2948=EDGE_CURVE('',#2318,#2319,#1852,.T.);
#2949=EDGE_CURVE('',#2320,#2319,#1853,.T.);
#2950=EDGE_CURVE('',#2320,#2321,#1854,.T.);
#2951=EDGE_CURVE('',#2062,#2321,#1855,.T.);
#2952=EDGE_CURVE('',#2322,#2061,#1856,.T.);
#2953=EDGE_CURVE('',#2322,#2323,#1857,.T.);
#2954=EDGE_CURVE('',#2324,#2323,#1858,.T.);
#2955=EDGE_CURVE('',#2324,#2325,#1859,.T.);
#2956=EDGE_CURVE('',#2058,#2325,#1860,.T.);
#2957=EDGE_CURVE('',#2326,#2057,#1861,.T.);
#2958=EDGE_CURVE('',#2326,#2327,#1862,.T.);
#2959=EDGE_CURVE('',#2328,#2327,#1863,.T.);
#2960=EDGE_CURVE('',#2328,#2329,#1864,.T.);
#2961=EDGE_CURVE('',#2046,#2329,#1865,.T.);
#2962=EDGE_CURVE('',#2330,#2045,#1866,.T.);
#2963=EDGE_CURVE('',#2330,#2331,#1867,.T.);
#2964=EDGE_CURVE('',#2332,#2331,#1868,.T.);
#2965=EDGE_CURVE('',#2332,#2240,#1869,.T.);
#2966=EDGE_CURVE('',#2333,#1969,#1030,.T.);
#2967=EDGE_CURVE('',#2334,#2333,#1031,.T.);
#2968=EDGE_CURVE('',#1970,#2334,#1032,.T.);
#2969=EDGE_CURVE('',#2257,#2221,#1033,.T.);
#2970=EDGE_CURVE('',#2225,#2253,#1034,.T.);
#2971=EDGE_CURVE('',#2256,#2222,#1035,.T.);
#2972=EDGE_CURVE('',#2254,#2224,#1036,.T.);
#2973=EDGE_CURVE('',#2223,#2255,#1037,.T.);
#2974=EDGE_CURVE('',#2252,#2226,#1038,.T.);
#2975=EDGE_CURVE('',#2229,#2249,#1039,.T.);
#2976=EDGE_CURVE('',#2250,#2228,#1040,.T.);
#2977=EDGE_CURVE('',#2227,#2251,#1041,.T.);
#2978=EDGE_CURVE('',#2204,#2274,#1042,.T.);
#2979=EDGE_CURVE('',#2275,#2203,#1043,.T.);
#2980=EDGE_CURVE('',#2202,#2276,#1044,.T.);
#2981=EDGE_CURVE('',#2277,#2201,#1045,.T.);
#2982=EDGE_CURVE('',#2198,#2280,#1046,.T.);
#2983=EDGE_CURVE('',#2281,#2197,#1047,.T.);
#2984=EDGE_CURVE('',#2200,#2278,#1048,.T.);
#2985=EDGE_CURVE('',#2279,#2199,#1049,.T.);
#2986=EDGE_CURVE('',#2206,#2272,#1050,.T.);
#2987=EDGE_CURVE('',#2273,#2205,#1051,.T.);
#2988=EDGE_CURVE('',#2271,#2207,#1052,.T.);
#2989=EDGE_CURVE('',#2208,#2270,#1053,.T.);
#2990=EDGE_CURVE('',#2269,#2209,#1054,.T.);
#2991=EDGE_CURVE('',#2210,#2268,#1055,.T.);
#2992=EDGE_CURVE('',#2267,#2211,#1056,.T.);
#2993=EDGE_CURVE('',#2212,#2266,#1057,.T.);
#2994=EDGE_CURVE('',#2263,#2215,#1058,.T.);
#2995=EDGE_CURVE('',#2216,#2262,#1059,.T.);
#2996=EDGE_CURVE('',#2265,#2213,#1060,.T.);
#2997=EDGE_CURVE('',#2214,#2264,#1061,.T.);
#2998=EDGE_CURVE('',#2261,#2217,#1062,.T.);
#2999=EDGE_CURVE('',#2218,#2260,#1063,.T.);
#3000=EDGE_CURVE('',#2259,#2219,#1064,.T.);
#3001=EDGE_CURVE('',#2220,#2258,#1065,.T.);
#3002=EDGE_CURVE('',#2196,#2282,#1066,.T.);
#3003=EDGE_CURVE('',#2283,#2195,#1067,.T.);
#3004=EDGE_CURVE('',#2194,#2284,#1068,.T.);
#3005=EDGE_CURVE('',#2285,#2193,#1069,.T.);
#3006=EDGE_CURVE('',#2289,#2189,#1070,.T.);
#3007=EDGE_CURVE('',#2192,#2286,#1071,.T.);
#3008=EDGE_CURVE('',#2287,#2191,#1072,.T.);
#3009=EDGE_CURVE('',#2190,#2288,#1073,.T.);
#3010=EDGE_CURVE('',#2293,#2185,#1074,.T.);
#3011=EDGE_CURVE('',#2188,#2290,#1075,.T.);
#3012=EDGE_CURVE('',#2291,#2187,#1076,.T.);
#3013=EDGE_CURVE('',#2186,#2292,#1077,.T.);
#3014=EDGE_CURVE('',#2305,#2173,#1078,.T.);
#3015=EDGE_CURVE('',#2176,#2302,#1079,.T.);
#3016=EDGE_CURVE('',#2303,#2175,#1080,.T.);
#3017=EDGE_CURVE('',#2174,#2304,#1081,.T.);
#3018=EDGE_CURVE('',#2309,#2169,#1082,.T.);
#3019=EDGE_CURVE('',#2172,#2306,#1083,.T.);
#3020=EDGE_CURVE('',#2307,#2171,#1084,.T.);
#3021=EDGE_CURVE('',#2170,#2308,#1085,.T.);
#3022=EDGE_CURVE('',#2301,#2177,#1086,.T.);
#3023=EDGE_CURVE('',#2180,#2298,#1087,.T.);
#3024=EDGE_CURVE('',#2299,#2179,#1088,.T.);
#3025=EDGE_CURVE('',#2178,#2300,#1089,.T.);
#3026=EDGE_CURVE('',#2297,#2181,#1090,.T.);
#3027=EDGE_CURVE('',#2184,#2294,#1091,.T.);
#3028=EDGE_CURVE('',#2295,#2183,#1092,.T.);
#3029=EDGE_CURVE('',#2182,#2296,#1093,.T.);
#3030=EDGE_CURVE('',#2313,#2165,#1094,.T.);
#3031=EDGE_CURVE('',#2168,#2310,#1095,.T.);
#3032=EDGE_CURVE('',#2311,#2167,#1096,.T.);
#3033=EDGE_CURVE('',#2166,#2312,#1097,.T.);
#3034=EDGE_CURVE('',#2317,#2161,#1098,.T.);
#3035=EDGE_CURVE('',#2164,#2314,#1099,.T.);
#3036=EDGE_CURVE('',#2315,#2163,#1100,.T.);
#3037=EDGE_CURVE('',#2162,#2316,#1101,.T.);
#3038=EDGE_CURVE('',#2321,#2157,#1102,.T.);
#3039=EDGE_CURVE('',#2160,#2318,#1103,.T.);
#3040=EDGE_CURVE('',#2319,#2159,#1104,.T.);
#3041=EDGE_CURVE('',#2158,#2320,#1105,.T.);
#3042=EDGE_CURVE('',#2325,#2153,#1106,.T.);
#3043=EDGE_CURVE('',#2156,#2322,#1107,.T.);
#3044=EDGE_CURVE('',#2323,#2155,#1108,.T.);
#3045=EDGE_CURVE('',#2154,#2324,#1109,.T.);
#3046=EDGE_CURVE('',#2248,#2230,#1110,.T.);
#3047=EDGE_CURVE('',#2233,#2245,#1111,.T.);
#3048=EDGE_CURVE('',#2246,#2232,#1112,.T.);
#3049=EDGE_CURVE('',#2231,#2247,#1113,.T.);
#3050=EDGE_CURVE('',#2244,#2234,#1114,.T.);
#3051=EDGE_CURVE('',#2237,#2241,#1115,.T.);
#3052=EDGE_CURVE('',#2242,#2236,#1116,.T.);
#3053=EDGE_CURVE('',#2235,#2243,#1117,.T.);
#3054=EDGE_CURVE('',#2329,#2149,#1118,.T.);
#3055=EDGE_CURVE('',#2152,#2326,#1119,.T.);
#3056=EDGE_CURVE('',#2327,#2151,#1120,.T.);
#3057=EDGE_CURVE('',#2150,#2328,#1121,.T.);
#3058=EDGE_CURVE('',#2240,#2145,#1122,.T.);
#3059=EDGE_CURVE('',#2148,#2330,#1123,.T.);
#3060=EDGE_CURVE('',#2331,#2147,#1124,.T.);
#3061=EDGE_CURVE('',#2146,#2332,#1125,.T.);
#3062=EDGE_CURVE('',#2238,#2334,#1126,.T.);
#3063=EDGE_CURVE('',#2239,#2333,#1127,.T.);
#3374=ORIENTED_EDGE('',*,*,#2512,.F.);
#3375=ORIENTED_EDGE('',*,*,#2513,.T.);
#3376=ORIENTED_EDGE('',*,*,#2514,.T.);
#3377=ORIENTED_EDGE('',*,*,#2515,.T.);
#3378=ORIENTED_EDGE('',*,*,#2516,.F.);
#3379=ORIENTED_EDGE('',*,*,#2517,.F.);
#3380=ORIENTED_EDGE('',*,*,#2518,.F.);
#3381=ORIENTED_EDGE('',*,*,#2519,.F.);
#3382=ORIENTED_EDGE('',*,*,#2520,.F.);
#3383=ORIENTED_EDGE('',*,*,#2521,.F.);
#3384=ORIENTED_EDGE('',*,*,#2522,.T.);
#3385=ORIENTED_EDGE('',*,*,#2519,.T.);
#3386=ORIENTED_EDGE('',*,*,#2523,.F.);
#3387=ORIENTED_EDGE('',*,*,#2524,.F.);
#3388=ORIENTED_EDGE('',*,*,#2525,.F.);
#3389=ORIENTED_EDGE('',*,*,#2526,.F.);
#3390=ORIENTED_EDGE('',*,*,#2527,.F.);
#3391=ORIENTED_EDGE('',*,*,#2528,.F.);
#3392=ORIENTED_EDGE('',*,*,#2529,.T.);
#3393=ORIENTED_EDGE('',*,*,#2526,.T.);
#3394=ORIENTED_EDGE('',*,*,#2530,.F.);
#3395=ORIENTED_EDGE('',*,*,#2531,.F.);
#3396=ORIENTED_EDGE('',*,*,#2532,.F.);
#3397=ORIENTED_EDGE('',*,*,#2533,.F.);
#3398=ORIENTED_EDGE('',*,*,#2534,.F.);
#3399=ORIENTED_EDGE('',*,*,#2531,.T.);
#3400=ORIENTED_EDGE('',*,*,#2535,.T.);
#3401=ORIENTED_EDGE('',*,*,#2536,.F.);
#3402=ORIENTED_EDGE('',*,*,#2537,.F.);
#3403=ORIENTED_EDGE('',*,*,#2538,.F.);
#3404=ORIENTED_EDGE('',*,*,#2539,.F.);
#3405=ORIENTED_EDGE('',*,*,#2540,.F.);
#3406=ORIENTED_EDGE('',*,*,#2541,.F.);
#3407=ORIENTED_EDGE('',*,*,#2538,.T.);
#3408=ORIENTED_EDGE('',*,*,#2542,.T.);
#3409=ORIENTED_EDGE('',*,*,#2543,.F.);
#3410=ORIENTED_EDGE('',*,*,#2544,.F.);
#3411=ORIENTED_EDGE('',*,*,#2545,.F.);
#3412=ORIENTED_EDGE('',*,*,#2546,.F.);
#3413=ORIENTED_EDGE('',*,*,#2547,.F.);
#3414=ORIENTED_EDGE('',*,*,#2548,.F.);
#3415=ORIENTED_EDGE('',*,*,#2549,.F.);
#3416=ORIENTED_EDGE('',*,*,#2550,.F.);
#3417=ORIENTED_EDGE('',*,*,#2551,.F.);
#3418=ORIENTED_EDGE('',*,*,#2552,.F.);
#3419=ORIENTED_EDGE('',*,*,#2553,.F.);
#3420=ORIENTED_EDGE('',*,*,#2554,.F.);
#3421=ORIENTED_EDGE('',*,*,#2555,.F.);
#3422=ORIENTED_EDGE('',*,*,#2556,.F.);
#3423=ORIENTED_EDGE('',*,*,#2557,.F.);
#3424=ORIENTED_EDGE('',*,*,#2558,.F.);
#3425=ORIENTED_EDGE('',*,*,#2559,.F.);
#3426=ORIENTED_EDGE('',*,*,#2560,.F.);
#3427=ORIENTED_EDGE('',*,*,#2561,.F.);
#3428=ORIENTED_EDGE('',*,*,#2562,.F.);
#3429=ORIENTED_EDGE('',*,*,#2563,.F.);
#3430=ORIENTED_EDGE('',*,*,#2564,.F.);
#3431=ORIENTED_EDGE('',*,*,#2565,.F.);
#3432=ORIENTED_EDGE('',*,*,#2566,.F.);
#3433=ORIENTED_EDGE('',*,*,#2567,.F.);
#3434=ORIENTED_EDGE('',*,*,#2568,.F.);
#3435=ORIENTED_EDGE('',*,*,#2569,.F.);
#3436=ORIENTED_EDGE('',*,*,#2570,.F.);
#3437=ORIENTED_EDGE('',*,*,#2571,.F.);
#3438=ORIENTED_EDGE('',*,*,#2572,.F.);
#3439=ORIENTED_EDGE('',*,*,#2573,.F.);
#3440=ORIENTED_EDGE('',*,*,#2574,.F.);
#3441=ORIENTED_EDGE('',*,*,#2575,.F.);
#3442=ORIENTED_EDGE('',*,*,#2576,.F.);
#3443=ORIENTED_EDGE('',*,*,#2577,.F.);
#3444=ORIENTED_EDGE('',*,*,#2578,.F.);
#3445=ORIENTED_EDGE('',*,*,#2579,.F.);
#3446=ORIENTED_EDGE('',*,*,#2580,.F.);
#3447=ORIENTED_EDGE('',*,*,#2581,.F.);
#3448=ORIENTED_EDGE('',*,*,#2582,.F.);
#3449=ORIENTED_EDGE('',*,*,#2583,.F.);
#3450=ORIENTED_EDGE('',*,*,#2584,.F.);
#3451=ORIENTED_EDGE('',*,*,#2585,.T.);
#3452=ORIENTED_EDGE('',*,*,#2586,.T.);
#3453=ORIENTED_EDGE('',*,*,#2587,.T.);
#3454=ORIENTED_EDGE('',*,*,#2588,.F.);
#3455=ORIENTED_EDGE('',*,*,#2589,.T.);
#3456=ORIENTED_EDGE('',*,*,#2590,.T.);
#3457=ORIENTED_EDGE('',*,*,#2591,.T.);
#3458=ORIENTED_EDGE('',*,*,#2592,.T.);
#3459=ORIENTED_EDGE('',*,*,#2593,.T.);
#3460=ORIENTED_EDGE('',*,*,#2594,.F.);
#3461=ORIENTED_EDGE('',*,*,#2595,.T.);
#3462=ORIENTED_EDGE('',*,*,#2596,.F.);
#3463=ORIENTED_EDGE('',*,*,#2597,.T.);
#3464=ORIENTED_EDGE('',*,*,#2598,.T.);
#3465=ORIENTED_EDGE('',*,*,#2599,.T.);
#3466=ORIENTED_EDGE('',*,*,#2600,.F.);
#3467=ORIENTED_EDGE('',*,*,#2601,.T.);
#3468=ORIENTED_EDGE('',*,*,#2602,.T.);
#3469=ORIENTED_EDGE('',*,*,#2603,.T.);
#3470=ORIENTED_EDGE('',*,*,#2604,.T.);
#3471=ORIENTED_EDGE('',*,*,#2605,.T.);
#3472=ORIENTED_EDGE('',*,*,#2606,.F.);
#3473=ORIENTED_EDGE('',*,*,#2607,.T.);
#3474=ORIENTED_EDGE('',*,*,#2608,.T.);
#3475=ORIENTED_EDGE('',*,*,#2609,.T.);
#3476=ORIENTED_EDGE('',*,*,#2610,.F.);
#3477=ORIENTED_EDGE('',*,*,#2611,.T.);
#3478=ORIENTED_EDGE('',*,*,#2612,.T.);
#3479=ORIENTED_EDGE('',*,*,#2613,.T.);
#3480=ORIENTED_EDGE('',*,*,#2614,.F.);
#3481=ORIENTED_EDGE('',*,*,#2615,.T.);
#3482=ORIENTED_EDGE('',*,*,#2616,.F.);
#3483=ORIENTED_EDGE('',*,*,#2617,.T.);
#3484=ORIENTED_EDGE('',*,*,#2618,.T.);
#3485=ORIENTED_EDGE('',*,*,#2619,.T.);
#3486=ORIENTED_EDGE('',*,*,#2620,.F.);
#3487=ORIENTED_EDGE('',*,*,#2621,.T.);
#3488=ORIENTED_EDGE('',*,*,#2622,.T.);
#3489=ORIENTED_EDGE('',*,*,#2623,.T.);
#3490=ORIENTED_EDGE('',*,*,#2624,.T.);
#3491=ORIENTED_EDGE('',*,*,#2625,.T.);
#3492=ORIENTED_EDGE('',*,*,#2626,.F.);
#3493=ORIENTED_EDGE('',*,*,#2627,.T.);
#3494=ORIENTED_EDGE('',*,*,#2628,.T.);
#3495=ORIENTED_EDGE('',*,*,#2629,.T.);
#3496=ORIENTED_EDGE('',*,*,#2630,.F.);
#3497=ORIENTED_EDGE('',*,*,#2631,.T.);
#3498=ORIENTED_EDGE('',*,*,#2632,.T.);
#3499=ORIENTED_EDGE('',*,*,#2633,.T.);
#3500=ORIENTED_EDGE('',*,*,#2634,.F.);
#3501=ORIENTED_EDGE('',*,*,#2635,.T.);
#3502=ORIENTED_EDGE('',*,*,#2636,.T.);
#3503=ORIENTED_EDGE('',*,*,#2637,.T.);
#3504=ORIENTED_EDGE('',*,*,#2638,.F.);
#3505=ORIENTED_EDGE('',*,*,#2639,.T.);
#3506=ORIENTED_EDGE('',*,*,#2640,.T.);
#3507=ORIENTED_EDGE('',*,*,#2641,.T.);
#3508=ORIENTED_EDGE('',*,*,#2642,.F.);
#3509=ORIENTED_EDGE('',*,*,#2521,.T.);
#3510=ORIENTED_EDGE('',*,*,#2643,.T.);
#3511=ORIENTED_EDGE('',*,*,#2644,.T.);
#3512=ORIENTED_EDGE('',*,*,#2645,.F.);
#3513=ORIENTED_EDGE('',*,*,#2528,.T.);
#3514=ORIENTED_EDGE('',*,*,#2646,.F.);
#3515=ORIENTED_EDGE('',*,*,#2647,.T.);
#3516=ORIENTED_EDGE('',*,*,#2648,.T.);
#3517=ORIENTED_EDGE('',*,*,#2543,.T.);
#3518=ORIENTED_EDGE('',*,*,#2649,.F.);
#3519=ORIENTED_EDGE('',*,*,#2650,.T.);
#3520=ORIENTED_EDGE('',*,*,#2651,.T.);
#3521=ORIENTED_EDGE('',*,*,#2652,.T.);
#3522=ORIENTED_EDGE('',*,*,#2653,.F.);
#3523=ORIENTED_EDGE('',*,*,#2654,.T.);
#3524=ORIENTED_EDGE('',*,*,#2655,.T.);
#3525=ORIENTED_EDGE('',*,*,#2656,.T.);
#3526=ORIENTED_EDGE('',*,*,#2657,.T.);
#3527=ORIENTED_EDGE('',*,*,#2658,.T.);
#3528=ORIENTED_EDGE('',*,*,#2659,.F.);
#3529=ORIENTED_EDGE('',*,*,#2660,.T.);
#3530=ORIENTED_EDGE('',*,*,#2661,.F.);
#3531=ORIENTED_EDGE('',*,*,#2662,.T.);
#3532=ORIENTED_EDGE('',*,*,#2663,.T.);
#3533=ORIENTED_EDGE('',*,*,#2664,.T.);
#3534=ORIENTED_EDGE('',*,*,#2665,.F.);
#3535=ORIENTED_EDGE('',*,*,#2666,.T.);
#3536=ORIENTED_EDGE('',*,*,#2667,.T.);
#3537=ORIENTED_EDGE('',*,*,#2668,.T.);
#3538=ORIENTED_EDGE('',*,*,#2669,.F.);
#3539=ORIENTED_EDGE('',*,*,#2670,.T.);
#3540=ORIENTED_EDGE('',*,*,#2671,.T.);
#3541=ORIENTED_EDGE('',*,*,#2672,.T.);
#3542=ORIENTED_EDGE('',*,*,#2673,.F.);
#3543=ORIENTED_EDGE('',*,*,#2674,.T.);
#3544=ORIENTED_EDGE('',*,*,#2675,.T.);
#3545=ORIENTED_EDGE('',*,*,#2676,.T.);
#3546=ORIENTED_EDGE('',*,*,#2677,.F.);
#3547=ORIENTED_EDGE('',*,*,#2678,.T.);
#3548=ORIENTED_EDGE('',*,*,#2679,.T.);
#3549=ORIENTED_EDGE('',*,*,#2680,.T.);
#3550=ORIENTED_EDGE('',*,*,#2681,.T.);
#3551=ORIENTED_EDGE('',*,*,#2682,.T.);
#3552=ORIENTED_EDGE('',*,*,#2683,.F.);
#3553=ORIENTED_EDGE('',*,*,#2684,.T.);
#3554=ORIENTED_EDGE('',*,*,#2685,.T.);
#3555=ORIENTED_EDGE('',*,*,#2686,.T.);
#3556=ORIENTED_EDGE('',*,*,#2687,.F.);
#3557=ORIENTED_EDGE('',*,*,#2688,.T.);
#3558=ORIENTED_EDGE('',*,*,#2689,.T.);
#3559=ORIENTED_EDGE('',*,*,#2690,.T.);
#3560=ORIENTED_EDGE('',*,*,#2691,.F.);
#3561=ORIENTED_EDGE('',*,*,#2692,.T.);
#3562=ORIENTED_EDGE('',*,*,#2693,.F.);
#3563=ORIENTED_EDGE('',*,*,#2694,.T.);
#3564=ORIENTED_EDGE('',*,*,#2695,.T.);
#3565=ORIENTED_EDGE('',*,*,#2696,.T.);
#3566=ORIENTED_EDGE('',*,*,#2590,.F.);
#3567=ORIENTED_EDGE('',*,*,#2697,.T.);
#3568=ORIENTED_EDGE('',*,*,#2698,.T.);
#3569=ORIENTED_EDGE('',*,*,#2699,.T.);
#3570=ORIENTED_EDGE('',*,*,#2700,.T.);
#3571=ORIENTED_EDGE('',*,*,#2701,.T.);
#3572=ORIENTED_EDGE('',*,*,#2592,.F.);
#3573=ORIENTED_EDGE('',*,*,#2702,.T.);
#3574=ORIENTED_EDGE('',*,*,#2703,.T.);
#3575=ORIENTED_EDGE('',*,*,#2704,.T.);
#3576=ORIENTED_EDGE('',*,*,#2705,.T.);
#3577=ORIENTED_EDGE('',*,*,#2706,.T.);
#3578=ORIENTED_EDGE('',*,*,#2604,.F.);
#3579=ORIENTED_EDGE('',*,*,#2707,.T.);
#3580=ORIENTED_EDGE('',*,*,#2708,.T.);
#3581=ORIENTED_EDGE('',*,*,#2709,.T.);
#3582=ORIENTED_EDGE('',*,*,#2710,.T.);
#3583=ORIENTED_EDGE('',*,*,#2711,.T.);
#3584=ORIENTED_EDGE('',*,*,#2608,.F.);
#3585=ORIENTED_EDGE('',*,*,#2712,.T.);
#3586=ORIENTED_EDGE('',*,*,#2713,.T.);
#3587=ORIENTED_EDGE('',*,*,#2714,.T.);
#3588=ORIENTED_EDGE('',*,*,#2715,.T.);
#3589=ORIENTED_EDGE('',*,*,#2716,.T.);
#3590=ORIENTED_EDGE('',*,*,#2586,.F.);
#3591=ORIENTED_EDGE('',*,*,#2717,.T.);
#3592=ORIENTED_EDGE('',*,*,#2718,.T.);
#3593=ORIENTED_EDGE('',*,*,#2719,.T.);
#3594=ORIENTED_EDGE('',*,*,#2720,.T.);
#3595=ORIENTED_EDGE('',*,*,#2721,.T.);
#3596=ORIENTED_EDGE('',*,*,#2612,.F.);
#3597=ORIENTED_EDGE('',*,*,#2722,.T.);
#3598=ORIENTED_EDGE('',*,*,#2723,.T.);
#3599=ORIENTED_EDGE('',*,*,#2724,.T.);
#3600=ORIENTED_EDGE('',*,*,#2725,.T.);
#3601=ORIENTED_EDGE('',*,*,#2726,.T.);
#3602=ORIENTED_EDGE('',*,*,#2624,.F.);
#3603=ORIENTED_EDGE('',*,*,#2727,.T.);
#3604=ORIENTED_EDGE('',*,*,#2728,.T.);
#3605=ORIENTED_EDGE('',*,*,#2729,.T.);
#3606=ORIENTED_EDGE('',*,*,#2730,.T.);
#3607=ORIENTED_EDGE('',*,*,#2731,.T.);
#3608=ORIENTED_EDGE('',*,*,#2628,.F.);
#3609=ORIENTED_EDGE('',*,*,#2732,.T.);
#3610=ORIENTED_EDGE('',*,*,#2733,.T.);
#3611=ORIENTED_EDGE('',*,*,#2734,.T.);
#3612=ORIENTED_EDGE('',*,*,#2735,.T.);
#3613=ORIENTED_EDGE('',*,*,#2736,.T.);
#3614=ORIENTED_EDGE('',*,*,#2622,.F.);
#3615=ORIENTED_EDGE('',*,*,#2737,.T.);
#3616=ORIENTED_EDGE('',*,*,#2738,.T.);
#3617=ORIENTED_EDGE('',*,*,#2739,.T.);
#3618=ORIENTED_EDGE('',*,*,#2740,.T.);
#3619=ORIENTED_EDGE('',*,*,#2741,.T.);
#3620=ORIENTED_EDGE('',*,*,#2618,.F.);
#3621=ORIENTED_EDGE('',*,*,#2742,.T.);
#3622=ORIENTED_EDGE('',*,*,#2743,.T.);
#3623=ORIENTED_EDGE('',*,*,#2744,.T.);
#3624=ORIENTED_EDGE('',*,*,#2745,.T.);
#3625=ORIENTED_EDGE('',*,*,#2746,.T.);
#3626=ORIENTED_EDGE('',*,*,#2632,.F.);
#3627=ORIENTED_EDGE('',*,*,#2747,.T.);
#3628=ORIENTED_EDGE('',*,*,#2748,.T.);
#3629=ORIENTED_EDGE('',*,*,#2749,.T.);
#3630=ORIENTED_EDGE('',*,*,#2750,.T.);
#3631=ORIENTED_EDGE('',*,*,#2751,.T.);
#3632=ORIENTED_EDGE('',*,*,#2636,.F.);
#3633=ORIENTED_EDGE('',*,*,#2752,.T.);
#3634=ORIENTED_EDGE('',*,*,#2753,.T.);
#3635=ORIENTED_EDGE('',*,*,#2754,.T.);
#3636=ORIENTED_EDGE('',*,*,#2755,.T.);
#3637=ORIENTED_EDGE('',*,*,#2756,.T.);
#3638=ORIENTED_EDGE('',*,*,#2640,.F.);
#3639=ORIENTED_EDGE('',*,*,#2520,.T.);
#3640=ORIENTED_EDGE('',*,*,#2518,.T.);
#3641=ORIENTED_EDGE('',*,*,#2757,.T.);
#3642=ORIENTED_EDGE('',*,*,#2758,.T.);
#3643=ORIENTED_EDGE('',*,*,#2759,.T.);
#3644=ORIENTED_EDGE('',*,*,#2643,.F.);
#3645=ORIENTED_EDGE('',*,*,#2527,.T.);
#3646=ORIENTED_EDGE('',*,*,#2525,.T.);
#3647=ORIENTED_EDGE('',*,*,#2760,.T.);
#3648=ORIENTED_EDGE('',*,*,#2761,.T.);
#3649=ORIENTED_EDGE('',*,*,#2762,.T.);
#3650=ORIENTED_EDGE('',*,*,#2681,.F.);
#3651=ORIENTED_EDGE('',*,*,#2763,.T.);
#3652=ORIENTED_EDGE('',*,*,#2574,.T.);
#3653=ORIENTED_EDGE('',*,*,#2764,.T.);
#3654=ORIENTED_EDGE('',*,*,#2765,.T.);
#3655=ORIENTED_EDGE('',*,*,#2766,.T.);
#3656=ORIENTED_EDGE('',*,*,#2679,.F.);
#3657=ORIENTED_EDGE('',*,*,#2767,.T.);
#3658=ORIENTED_EDGE('',*,*,#2570,.T.);
#3659=ORIENTED_EDGE('',*,*,#2768,.T.);
#3660=ORIENTED_EDGE('',*,*,#2769,.T.);
#3661=ORIENTED_EDGE('',*,*,#2770,.T.);
#3662=ORIENTED_EDGE('',*,*,#2685,.F.);
#3663=ORIENTED_EDGE('',*,*,#2771,.T.);
#3664=ORIENTED_EDGE('',*,*,#2578,.T.);
#3665=ORIENTED_EDGE('',*,*,#2772,.T.);
#3666=ORIENTED_EDGE('',*,*,#2773,.T.);
#3667=ORIENTED_EDGE('',*,*,#2774,.T.);
#3668=ORIENTED_EDGE('',*,*,#2689,.F.);
#3669=ORIENTED_EDGE('',*,*,#2775,.T.);
#3670=ORIENTED_EDGE('',*,*,#2582,.T.);
#3671=ORIENTED_EDGE('',*,*,#2776,.T.);
#3672=ORIENTED_EDGE('',*,*,#2777,.T.);
#3673=ORIENTED_EDGE('',*,*,#2778,.T.);
#3674=ORIENTED_EDGE('',*,*,#2675,.F.);
#3675=ORIENTED_EDGE('',*,*,#2779,.T.);
#3676=ORIENTED_EDGE('',*,*,#2566,.T.);
#3677=ORIENTED_EDGE('',*,*,#2780,.T.);
#3678=ORIENTED_EDGE('',*,*,#2781,.T.);
#3679=ORIENTED_EDGE('',*,*,#2782,.T.);
#3680=ORIENTED_EDGE('',*,*,#2671,.F.);
#3681=ORIENTED_EDGE('',*,*,#2783,.T.);
#3682=ORIENTED_EDGE('',*,*,#2784,.T.);
#3683=ORIENTED_EDGE('',*,*,#2785,.T.);
#3684=ORIENTED_EDGE('',*,*,#2562,.T.);
#3685=ORIENTED_EDGE('',*,*,#2786,.T.);
#3686=ORIENTED_EDGE('',*,*,#2667,.F.);
#3687=ORIENTED_EDGE('',*,*,#2787,.T.);
#3688=ORIENTED_EDGE('',*,*,#2788,.T.);
#3689=ORIENTED_EDGE('',*,*,#2789,.T.);
#3690=ORIENTED_EDGE('',*,*,#2558,.T.);
#3691=ORIENTED_EDGE('',*,*,#2790,.T.);
#3692=ORIENTED_EDGE('',*,*,#2663,.F.);
#3693=ORIENTED_EDGE('',*,*,#2791,.T.);
#3694=ORIENTED_EDGE('',*,*,#2792,.T.);
#3695=ORIENTED_EDGE('',*,*,#2793,.T.);
#3696=ORIENTED_EDGE('',*,*,#2554,.T.);
#3697=ORIENTED_EDGE('',*,*,#2794,.T.);
#3698=ORIENTED_EDGE('',*,*,#2655,.F.);
#3699=ORIENTED_EDGE('',*,*,#2795,.T.);
#3700=ORIENTED_EDGE('',*,*,#2796,.T.);
#3701=ORIENTED_EDGE('',*,*,#2797,.T.);
#3702=ORIENTED_EDGE('',*,*,#2546,.T.);
#3703=ORIENTED_EDGE('',*,*,#2798,.T.);
#3704=ORIENTED_EDGE('',*,*,#2657,.F.);
#3705=ORIENTED_EDGE('',*,*,#2799,.T.);
#3706=ORIENTED_EDGE('',*,*,#2800,.T.);
#3707=ORIENTED_EDGE('',*,*,#2801,.T.);
#3708=ORIENTED_EDGE('',*,*,#2550,.T.);
#3709=ORIENTED_EDGE('',*,*,#2802,.T.);
#3710=ORIENTED_EDGE('',*,*,#2651,.F.);
#3711=ORIENTED_EDGE('',*,*,#2803,.T.);
#3712=ORIENTED_EDGE('',*,*,#2804,.T.);
#3713=ORIENTED_EDGE('',*,*,#2805,.T.);
#3714=ORIENTED_EDGE('',*,*,#2539,.T.);
#3715=ORIENTED_EDGE('',*,*,#2541,.T.);
#3716=ORIENTED_EDGE('',*,*,#2648,.F.);
#3717=ORIENTED_EDGE('',*,*,#2806,.T.);
#3718=ORIENTED_EDGE('',*,*,#2807,.T.);
#3719=ORIENTED_EDGE('',*,*,#2808,.T.);
#3720=ORIENTED_EDGE('',*,*,#2532,.T.);
#3721=ORIENTED_EDGE('',*,*,#2534,.T.);
#3722=ORIENTED_EDGE('',*,*,#2809,.F.);
#3723=ORIENTED_EDGE('',*,*,#2810,.T.);
#3724=ORIENTED_EDGE('',*,*,#2811,.T.);
#3725=ORIENTED_EDGE('',*,*,#2812,.T.);
#3726=ORIENTED_EDGE('',*,*,#2813,.T.);
#3727=ORIENTED_EDGE('',*,*,#2814,.T.);
#3728=ORIENTED_EDGE('',*,*,#2695,.F.);
#3729=ORIENTED_EDGE('',*,*,#2815,.T.);
#3730=ORIENTED_EDGE('',*,*,#2816,.T.);
#3731=ORIENTED_EDGE('',*,*,#2817,.T.);
#3732=ORIENTED_EDGE('',*,*,#2818,.T.);
#3733=ORIENTED_EDGE('',*,*,#2819,.T.);
#3734=ORIENTED_EDGE('',*,*,#2602,.F.);
#3735=ORIENTED_EDGE('',*,*,#2820,.T.);
#3736=ORIENTED_EDGE('',*,*,#2821,.T.);
#3737=ORIENTED_EDGE('',*,*,#2822,.T.);
#3738=ORIENTED_EDGE('',*,*,#2823,.T.);
#3739=ORIENTED_EDGE('',*,*,#2824,.T.);
#3740=ORIENTED_EDGE('',*,*,#2598,.F.);
#3741=ORIENTED_EDGE('',*,*,#2825,.T.);
#3742=ORIENTED_EDGE('',*,*,#2826,.T.);
#3743=ORIENTED_EDGE('',*,*,#2827,.T.);
#3744=ORIENTED_EDGE('',*,*,#2828,.T.);
#3745=ORIENTED_EDGE('',*,*,#2829,.T.);
#3746=ORIENTED_EDGE('',*,*,#2830,.T.);
#3747=ORIENTED_EDGE('',*,*,#2831,.T.);
#3748=ORIENTED_EDGE('',*,*,#2512,.T.);
#3749=ORIENTED_EDGE('',*,*,#2832,.T.);
#3750=ORIENTED_EDGE('',*,*,#2833,.F.);
#3751=ORIENTED_EDGE('',*,*,#2588,.T.);
#3752=ORIENTED_EDGE('',*,*,#2834,.F.);
#3753=ORIENTED_EDGE('',*,*,#2835,.T.);
#3754=ORIENTED_EDGE('',*,*,#2836,.F.);
#3755=ORIENTED_EDGE('',*,*,#2837,.T.);
#3756=ORIENTED_EDGE('',*,*,#2838,.F.);
#3757=ORIENTED_EDGE('',*,*,#2596,.T.);
#3758=ORIENTED_EDGE('',*,*,#2839,.F.);
#3759=ORIENTED_EDGE('',*,*,#2840,.T.);
#3760=ORIENTED_EDGE('',*,*,#2841,.F.);
#3761=ORIENTED_EDGE('',*,*,#2842,.T.);
#3762=ORIENTED_EDGE('',*,*,#2843,.F.);
#3763=ORIENTED_EDGE('',*,*,#2600,.T.);
#3764=ORIENTED_EDGE('',*,*,#2844,.F.);
#3765=ORIENTED_EDGE('',*,*,#2845,.T.);
#3766=ORIENTED_EDGE('',*,*,#2846,.F.);
#3767=ORIENTED_EDGE('',*,*,#2847,.T.);
#3768=ORIENTED_EDGE('',*,*,#2848,.F.);
#3769=ORIENTED_EDGE('',*,*,#2693,.T.);
#3770=ORIENTED_EDGE('',*,*,#2849,.F.);
#3771=ORIENTED_EDGE('',*,*,#2850,.T.);
#3772=ORIENTED_EDGE('',*,*,#2851,.F.);
#3773=ORIENTED_EDGE('',*,*,#2852,.T.);
#3774=ORIENTED_EDGE('',*,*,#2853,.F.);
#3775=ORIENTED_EDGE('',*,*,#2854,.T.);
#3776=ORIENTED_EDGE('',*,*,#2535,.F.);
#3777=ORIENTED_EDGE('',*,*,#2530,.T.);
#3778=ORIENTED_EDGE('',*,*,#2855,.F.);
#3779=ORIENTED_EDGE('',*,*,#2856,.T.);
#3780=ORIENTED_EDGE('',*,*,#2857,.F.);
#3781=ORIENTED_EDGE('',*,*,#2646,.T.);
#3782=ORIENTED_EDGE('',*,*,#2542,.F.);
#3783=ORIENTED_EDGE('',*,*,#2537,.T.);
#3784=ORIENTED_EDGE('',*,*,#2858,.F.);
#3785=ORIENTED_EDGE('',*,*,#2859,.T.);
#3786=ORIENTED_EDGE('',*,*,#2860,.F.);
#3787=ORIENTED_EDGE('',*,*,#2649,.T.);
#3788=ORIENTED_EDGE('',*,*,#2861,.F.);
#3789=ORIENTED_EDGE('',*,*,#2548,.T.);
#3790=ORIENTED_EDGE('',*,*,#2862,.F.);
#3791=ORIENTED_EDGE('',*,*,#2863,.T.);
#3792=ORIENTED_EDGE('',*,*,#2864,.F.);
#3793=ORIENTED_EDGE('',*,*,#2659,.T.);
#3794=ORIENTED_EDGE('',*,*,#2865,.F.);
#3795=ORIENTED_EDGE('',*,*,#2544,.T.);
#3796=ORIENTED_EDGE('',*,*,#2866,.F.);
#3797=ORIENTED_EDGE('',*,*,#2867,.T.);
#3798=ORIENTED_EDGE('',*,*,#2868,.F.);
#3799=ORIENTED_EDGE('',*,*,#2653,.T.);
#3800=ORIENTED_EDGE('',*,*,#2869,.F.);
#3801=ORIENTED_EDGE('',*,*,#2552,.T.);
#3802=ORIENTED_EDGE('',*,*,#2870,.F.);
#3803=ORIENTED_EDGE('',*,*,#2871,.T.);
#3804=ORIENTED_EDGE('',*,*,#2872,.F.);
#3805=ORIENTED_EDGE('',*,*,#2661,.T.);
#3806=ORIENTED_EDGE('',*,*,#2873,.F.);
#3807=ORIENTED_EDGE('',*,*,#2556,.T.);
#3808=ORIENTED_EDGE('',*,*,#2874,.F.);
#3809=ORIENTED_EDGE('',*,*,#2875,.T.);
#3810=ORIENTED_EDGE('',*,*,#2876,.F.);
#3811=ORIENTED_EDGE('',*,*,#2665,.T.);
#3812=ORIENTED_EDGE('',*,*,#2877,.F.);
#3813=ORIENTED_EDGE('',*,*,#2560,.T.);
#3814=ORIENTED_EDGE('',*,*,#2878,.F.);
#3815=ORIENTED_EDGE('',*,*,#2879,.T.);
#3816=ORIENTED_EDGE('',*,*,#2880,.F.);
#3817=ORIENTED_EDGE('',*,*,#2669,.T.);
#3818=ORIENTED_EDGE('',*,*,#2881,.F.);
#3819=ORIENTED_EDGE('',*,*,#2882,.T.);
#3820=ORIENTED_EDGE('',*,*,#2883,.F.);
#3821=ORIENTED_EDGE('',*,*,#2564,.T.);
#3822=ORIENTED_EDGE('',*,*,#2884,.F.);
#3823=ORIENTED_EDGE('',*,*,#2673,.T.);
#3824=ORIENTED_EDGE('',*,*,#2885,.F.);
#3825=ORIENTED_EDGE('',*,*,#2886,.T.);
#3826=ORIENTED_EDGE('',*,*,#2887,.F.);
#3827=ORIENTED_EDGE('',*,*,#2580,.T.);
#3828=ORIENTED_EDGE('',*,*,#2888,.F.);
#3829=ORIENTED_EDGE('',*,*,#2691,.T.);
#3830=ORIENTED_EDGE('',*,*,#2889,.F.);
#3831=ORIENTED_EDGE('',*,*,#2890,.T.);
#3832=ORIENTED_EDGE('',*,*,#2891,.F.);
#3833=ORIENTED_EDGE('',*,*,#2576,.T.);
#3834=ORIENTED_EDGE('',*,*,#2892,.F.);
#3835=ORIENTED_EDGE('',*,*,#2687,.T.);
#3836=ORIENTED_EDGE('',*,*,#2893,.F.);
#3837=ORIENTED_EDGE('',*,*,#2894,.T.);
#3838=ORIENTED_EDGE('',*,*,#2895,.F.);
#3839=ORIENTED_EDGE('',*,*,#2568,.T.);
#3840=ORIENTED_EDGE('',*,*,#2896,.F.);
#3841=ORIENTED_EDGE('',*,*,#2677,.T.);
#3842=ORIENTED_EDGE('',*,*,#2897,.F.);
#3843=ORIENTED_EDGE('',*,*,#2898,.T.);
#3844=ORIENTED_EDGE('',*,*,#2899,.F.);
#3845=ORIENTED_EDGE('',*,*,#2572,.T.);
#3846=ORIENTED_EDGE('',*,*,#2900,.F.);
#3847=ORIENTED_EDGE('',*,*,#2683,.T.);
#3848=ORIENTED_EDGE('',*,*,#2901,.F.);
#3849=ORIENTED_EDGE('',*,*,#2902,.T.);
#3850=ORIENTED_EDGE('',*,*,#2903,.F.);
#3851=ORIENTED_EDGE('',*,*,#2523,.T.);
#3852=ORIENTED_EDGE('',*,*,#2529,.F.);
#3853=ORIENTED_EDGE('',*,*,#2645,.T.);
#3854=ORIENTED_EDGE('',*,*,#2904,.F.);
#3855=ORIENTED_EDGE('',*,*,#2905,.T.);
#3856=ORIENTED_EDGE('',*,*,#2906,.F.);
#3857=ORIENTED_EDGE('',*,*,#2516,.T.);
#3858=ORIENTED_EDGE('',*,*,#2522,.F.);
#3859=ORIENTED_EDGE('',*,*,#2642,.T.);
#3860=ORIENTED_EDGE('',*,*,#2907,.F.);
#3861=ORIENTED_EDGE('',*,*,#2908,.T.);
#3862=ORIENTED_EDGE('',*,*,#2909,.F.);
#3863=ORIENTED_EDGE('',*,*,#2910,.T.);
#3864=ORIENTED_EDGE('',*,*,#2911,.F.);
#3865=ORIENTED_EDGE('',*,*,#2638,.T.);
#3866=ORIENTED_EDGE('',*,*,#2912,.F.);
#3867=ORIENTED_EDGE('',*,*,#2913,.T.);
#3868=ORIENTED_EDGE('',*,*,#2914,.F.);
#3869=ORIENTED_EDGE('',*,*,#2915,.T.);
#3870=ORIENTED_EDGE('',*,*,#2916,.F.);
#3871=ORIENTED_EDGE('',*,*,#2634,.T.);
#3872=ORIENTED_EDGE('',*,*,#2917,.F.);
#3873=ORIENTED_EDGE('',*,*,#2918,.T.);
#3874=ORIENTED_EDGE('',*,*,#2919,.F.);
#3875=ORIENTED_EDGE('',*,*,#2920,.T.);
#3876=ORIENTED_EDGE('',*,*,#2921,.F.);
#3877=ORIENTED_EDGE('',*,*,#2616,.T.);
#3878=ORIENTED_EDGE('',*,*,#2922,.F.);
#3879=ORIENTED_EDGE('',*,*,#2923,.T.);
#3880=ORIENTED_EDGE('',*,*,#2924,.F.);
#3881=ORIENTED_EDGE('',*,*,#2925,.T.);
#3882=ORIENTED_EDGE('',*,*,#2926,.F.);
#3883=ORIENTED_EDGE('',*,*,#2620,.T.);
#3884=ORIENTED_EDGE('',*,*,#2927,.F.);
#3885=ORIENTED_EDGE('',*,*,#2928,.T.);
#3886=ORIENTED_EDGE('',*,*,#2929,.F.);
#3887=ORIENTED_EDGE('',*,*,#2930,.T.);
#3888=ORIENTED_EDGE('',*,*,#2931,.F.);
#3889=ORIENTED_EDGE('',*,*,#2630,.T.);
#3890=ORIENTED_EDGE('',*,*,#2932,.F.);
#3891=ORIENTED_EDGE('',*,*,#2933,.T.);
#3892=ORIENTED_EDGE('',*,*,#2934,.F.);
#3893=ORIENTED_EDGE('',*,*,#2935,.T.);
#3894=ORIENTED_EDGE('',*,*,#2936,.F.);
#3895=ORIENTED_EDGE('',*,*,#2626,.T.);
#3896=ORIENTED_EDGE('',*,*,#2937,.F.);
#3897=ORIENTED_EDGE('',*,*,#2938,.T.);
#3898=ORIENTED_EDGE('',*,*,#2939,.F.);
#3899=ORIENTED_EDGE('',*,*,#2940,.T.);
#3900=ORIENTED_EDGE('',*,*,#2941,.F.);
#3901=ORIENTED_EDGE('',*,*,#2614,.T.);
#3902=ORIENTED_EDGE('',*,*,#2942,.F.);
#3903=ORIENTED_EDGE('',*,*,#2943,.T.);
#3904=ORIENTED_EDGE('',*,*,#2944,.F.);
#3905=ORIENTED_EDGE('',*,*,#2945,.T.);
#3906=ORIENTED_EDGE('',*,*,#2946,.F.);
#3907=ORIENTED_EDGE('',*,*,#2584,.T.);
#3908=ORIENTED_EDGE('',*,*,#2947,.F.);
#3909=ORIENTED_EDGE('',*,*,#2948,.T.);
#3910=ORIENTED_EDGE('',*,*,#2949,.F.);
#3911=ORIENTED_EDGE('',*,*,#2950,.T.);
#3912=ORIENTED_EDGE('',*,*,#2951,.F.);
#3913=ORIENTED_EDGE('',*,*,#2610,.T.);
#3914=ORIENTED_EDGE('',*,*,#2952,.F.);
#3915=ORIENTED_EDGE('',*,*,#2953,.T.);
#3916=ORIENTED_EDGE('',*,*,#2954,.F.);
#3917=ORIENTED_EDGE('',*,*,#2955,.T.);
#3918=ORIENTED_EDGE('',*,*,#2956,.F.);
#3919=ORIENTED_EDGE('',*,*,#2606,.T.);
#3920=ORIENTED_EDGE('',*,*,#2957,.F.);
#3921=ORIENTED_EDGE('',*,*,#2958,.T.);
#3922=ORIENTED_EDGE('',*,*,#2959,.F.);
#3923=ORIENTED_EDGE('',*,*,#2960,.T.);
#3924=ORIENTED_EDGE('',*,*,#2961,.F.);
#3925=ORIENTED_EDGE('',*,*,#2594,.T.);
#3926=ORIENTED_EDGE('',*,*,#2962,.F.);
#3927=ORIENTED_EDGE('',*,*,#2963,.T.);
#3928=ORIENTED_EDGE('',*,*,#2964,.F.);
#3929=ORIENTED_EDGE('',*,*,#2965,.T.);
#3930=ORIENTED_EDGE('',*,*,#2966,.F.);
#3931=ORIENTED_EDGE('',*,*,#2967,.F.);
#3932=ORIENTED_EDGE('',*,*,#2968,.F.);
#3933=ORIENTED_EDGE('',*,*,#2514,.F.);
#3934=ORIENTED_EDGE('',*,*,#2809,.T.);
#3935=ORIENTED_EDGE('',*,*,#2536,.T.);
#3936=ORIENTED_EDGE('',*,*,#2854,.F.);
#3937=ORIENTED_EDGE('',*,*,#2969,.T.);
#3938=ORIENTED_EDGE('',*,*,#2814,.F.);
#3939=ORIENTED_EDGE('',*,*,#2970,.T.);
#3940=ORIENTED_EDGE('',*,*,#2849,.T.);
#3941=ORIENTED_EDGE('',*,*,#2696,.F.);
#3942=ORIENTED_EDGE('',*,*,#2853,.T.);
#3943=ORIENTED_EDGE('',*,*,#2971,.T.);
#3944=ORIENTED_EDGE('',*,*,#2810,.F.);
#3945=ORIENTED_EDGE('',*,*,#2969,.F.);
#3946=ORIENTED_EDGE('',*,*,#2851,.T.);
#3947=ORIENTED_EDGE('',*,*,#2972,.T.);
#3948=ORIENTED_EDGE('',*,*,#2812,.F.);
#3949=ORIENTED_EDGE('',*,*,#2973,.T.);
#3950=ORIENTED_EDGE('',*,*,#2813,.F.);
#3951=ORIENTED_EDGE('',*,*,#2972,.F.);
#3952=ORIENTED_EDGE('',*,*,#2850,.F.);
#3953=ORIENTED_EDGE('',*,*,#2970,.F.);
#3954=ORIENTED_EDGE('',*,*,#2811,.F.);
#3955=ORIENTED_EDGE('',*,*,#2971,.F.);
#3956=ORIENTED_EDGE('',*,*,#2852,.F.);
#3957=ORIENTED_EDGE('',*,*,#2973,.F.);
#3958=ORIENTED_EDGE('',*,*,#2848,.T.);
#3959=ORIENTED_EDGE('',*,*,#2974,.T.);
#3960=ORIENTED_EDGE('',*,*,#2815,.F.);
#3961=ORIENTED_EDGE('',*,*,#2694,.F.);
#3962=ORIENTED_EDGE('',*,*,#2819,.F.);
#3963=ORIENTED_EDGE('',*,*,#2975,.T.);
#3964=ORIENTED_EDGE('',*,*,#2844,.T.);
#3965=ORIENTED_EDGE('',*,*,#2603,.F.);
#3966=ORIENTED_EDGE('',*,*,#2818,.F.);
#3967=ORIENTED_EDGE('',*,*,#2976,.F.);
#3968=ORIENTED_EDGE('',*,*,#2845,.F.);
#3969=ORIENTED_EDGE('',*,*,#2975,.F.);
#3970=ORIENTED_EDGE('',*,*,#2846,.T.);
#3971=ORIENTED_EDGE('',*,*,#2976,.T.);
#3972=ORIENTED_EDGE('',*,*,#2817,.F.);
#3973=ORIENTED_EDGE('',*,*,#2977,.T.);
#3974=ORIENTED_EDGE('',*,*,#2816,.F.);
#3975=ORIENTED_EDGE('',*,*,#2974,.F.);
#3976=ORIENTED_EDGE('',*,*,#2847,.F.);
#3977=ORIENTED_EDGE('',*,*,#2977,.F.);
#3978=ORIENTED_EDGE('',*,*,#2888,.T.);
#3979=ORIENTED_EDGE('',*,*,#2583,.T.);
#3980=ORIENTED_EDGE('',*,*,#2775,.F.);
#3981=ORIENTED_EDGE('',*,*,#2692,.F.);
#3982=ORIENTED_EDGE('',*,*,#2778,.F.);
#3983=ORIENTED_EDGE('',*,*,#2978,.T.);
#3984=ORIENTED_EDGE('',*,*,#2885,.T.);
#3985=ORIENTED_EDGE('',*,*,#2676,.F.);
#3986=ORIENTED_EDGE('',*,*,#2777,.F.);
#3987=ORIENTED_EDGE('',*,*,#2979,.F.);
#3988=ORIENTED_EDGE('',*,*,#2886,.F.);
#3989=ORIENTED_EDGE('',*,*,#2978,.F.);
#3990=ORIENTED_EDGE('',*,*,#2887,.T.);
#3991=ORIENTED_EDGE('',*,*,#2979,.T.);
#3992=ORIENTED_EDGE('',*,*,#2776,.F.);
#3993=ORIENTED_EDGE('',*,*,#2581,.T.);
#3994=ORIENTED_EDGE('',*,*,#2892,.T.);
#3995=ORIENTED_EDGE('',*,*,#2579,.T.);
#3996=ORIENTED_EDGE('',*,*,#2771,.F.);
#3997=ORIENTED_EDGE('',*,*,#2688,.F.);
#3998=ORIENTED_EDGE('',*,*,#2774,.F.);
#3999=ORIENTED_EDGE('',*,*,#2980,.T.);
#4000=ORIENTED_EDGE('',*,*,#2889,.T.);
#4001=ORIENTED_EDGE('',*,*,#2690,.F.);
#4002=ORIENTED_EDGE('',*,*,#2773,.F.);
#4003=ORIENTED_EDGE('',*,*,#2981,.F.);
#4004=ORIENTED_EDGE('',*,*,#2890,.F.);
#4005=ORIENTED_EDGE('',*,*,#2980,.F.);
#4006=ORIENTED_EDGE('',*,*,#2891,.T.);
#4007=ORIENTED_EDGE('',*,*,#2981,.T.);
#4008=ORIENTED_EDGE('',*,*,#2772,.F.);
#4009=ORIENTED_EDGE('',*,*,#2577,.T.);
#4010=ORIENTED_EDGE('',*,*,#2900,.T.);
#4011=ORIENTED_EDGE('',*,*,#2575,.T.);
#4012=ORIENTED_EDGE('',*,*,#2763,.F.);
#4013=ORIENTED_EDGE('',*,*,#2684,.F.);
#4014=ORIENTED_EDGE('',*,*,#2766,.F.);
#4015=ORIENTED_EDGE('',*,*,#2982,.T.);
#4016=ORIENTED_EDGE('',*,*,#2897,.T.);
#4017=ORIENTED_EDGE('',*,*,#2680,.F.);
#4018=ORIENTED_EDGE('',*,*,#2765,.F.);
#4019=ORIENTED_EDGE('',*,*,#2983,.F.);
#4020=ORIENTED_EDGE('',*,*,#2898,.F.);
#4021=ORIENTED_EDGE('',*,*,#2982,.F.);
#4022=ORIENTED_EDGE('',*,*,#2899,.T.);
#4023=ORIENTED_EDGE('',*,*,#2983,.T.);
#4024=ORIENTED_EDGE('',*,*,#2764,.F.);
#4025=ORIENTED_EDGE('',*,*,#2573,.T.);
#4026=ORIENTED_EDGE('',*,*,#2896,.T.);
#4027=ORIENTED_EDGE('',*,*,#2571,.T.);
#4028=ORIENTED_EDGE('',*,*,#2767,.F.);
#4029=ORIENTED_EDGE('',*,*,#2678,.F.);
#4030=ORIENTED_EDGE('',*,*,#2770,.F.);
#4031=ORIENTED_EDGE('',*,*,#2984,.T.);
#4032=ORIENTED_EDGE('',*,*,#2893,.T.);
#4033=ORIENTED_EDGE('',*,*,#2686,.F.);
#4034=ORIENTED_EDGE('',*,*,#2769,.F.);
#4035=ORIENTED_EDGE('',*,*,#2985,.F.);
#4036=ORIENTED_EDGE('',*,*,#2894,.F.);
#4037=ORIENTED_EDGE('',*,*,#2984,.F.);
#4038=ORIENTED_EDGE('',*,*,#2895,.T.);
#4039=ORIENTED_EDGE('',*,*,#2985,.T.);
#4040=ORIENTED_EDGE('',*,*,#2768,.F.);
#4041=ORIENTED_EDGE('',*,*,#2569,.T.);
#4042=ORIENTED_EDGE('',*,*,#2884,.T.);
#4043=ORIENTED_EDGE('',*,*,#2567,.T.);
#4044=ORIENTED_EDGE('',*,*,#2779,.F.);
#4045=ORIENTED_EDGE('',*,*,#2674,.F.);
#4046=ORIENTED_EDGE('',*,*,#2782,.F.);
#4047=ORIENTED_EDGE('',*,*,#2986,.T.);
#4048=ORIENTED_EDGE('',*,*,#2881,.T.);
#4049=ORIENTED_EDGE('',*,*,#2672,.F.);
#4050=ORIENTED_EDGE('',*,*,#2781,.F.);
#4051=ORIENTED_EDGE('',*,*,#2987,.F.);
#4052=ORIENTED_EDGE('',*,*,#2882,.F.);
#4053=ORIENTED_EDGE('',*,*,#2986,.F.);
#4054=ORIENTED_EDGE('',*,*,#2883,.T.);
#4055=ORIENTED_EDGE('',*,*,#2987,.T.);
#4056=ORIENTED_EDGE('',*,*,#2780,.F.);
#4057=ORIENTED_EDGE('',*,*,#2565,.T.);
#4058=ORIENTED_EDGE('',*,*,#2880,.T.);
#4059=ORIENTED_EDGE('',*,*,#2988,.T.);
#4060=ORIENTED_EDGE('',*,*,#2783,.F.);
#4061=ORIENTED_EDGE('',*,*,#2670,.F.);
#4062=ORIENTED_EDGE('',*,*,#2786,.F.);
#4063=ORIENTED_EDGE('',*,*,#2561,.T.);
#4064=ORIENTED_EDGE('',*,*,#2877,.T.);
#4065=ORIENTED_EDGE('',*,*,#2668,.F.);
#4066=ORIENTED_EDGE('',*,*,#2878,.T.);
#4067=ORIENTED_EDGE('',*,*,#2563,.T.);
#4068=ORIENTED_EDGE('',*,*,#2785,.F.);
#4069=ORIENTED_EDGE('',*,*,#2989,.T.);
#4070=ORIENTED_EDGE('',*,*,#2784,.F.);
#4071=ORIENTED_EDGE('',*,*,#2988,.F.);
#4072=ORIENTED_EDGE('',*,*,#2879,.F.);
#4073=ORIENTED_EDGE('',*,*,#2989,.F.);
#4074=ORIENTED_EDGE('',*,*,#2876,.T.);
#4075=ORIENTED_EDGE('',*,*,#2990,.T.);
#4076=ORIENTED_EDGE('',*,*,#2787,.F.);
#4077=ORIENTED_EDGE('',*,*,#2666,.F.);
#4078=ORIENTED_EDGE('',*,*,#2790,.F.);
#4079=ORIENTED_EDGE('',*,*,#2557,.T.);
#4080=ORIENTED_EDGE('',*,*,#2873,.T.);
#4081=ORIENTED_EDGE('',*,*,#2664,.F.);
#4082=ORIENTED_EDGE('',*,*,#2874,.T.);
#4083=ORIENTED_EDGE('',*,*,#2559,.T.);
#4084=ORIENTED_EDGE('',*,*,#2789,.F.);
#4085=ORIENTED_EDGE('',*,*,#2991,.T.);
#4086=ORIENTED_EDGE('',*,*,#2788,.F.);
#4087=ORIENTED_EDGE('',*,*,#2990,.F.);
#4088=ORIENTED_EDGE('',*,*,#2875,.F.);
#4089=ORIENTED_EDGE('',*,*,#2991,.F.);
#4090=ORIENTED_EDGE('',*,*,#2872,.T.);
#4091=ORIENTED_EDGE('',*,*,#2992,.T.);
#4092=ORIENTED_EDGE('',*,*,#2791,.F.);
#4093=ORIENTED_EDGE('',*,*,#2662,.F.);
#4094=ORIENTED_EDGE('',*,*,#2794,.F.);
#4095=ORIENTED_EDGE('',*,*,#2553,.T.);
#4096=ORIENTED_EDGE('',*,*,#2869,.T.);
#4097=ORIENTED_EDGE('',*,*,#2656,.F.);
#4098=ORIENTED_EDGE('',*,*,#2870,.T.);
#4099=ORIENTED_EDGE('',*,*,#2555,.T.);
#4100=ORIENTED_EDGE('',*,*,#2793,.F.);
#4101=ORIENTED_EDGE('',*,*,#2993,.T.);
#4102=ORIENTED_EDGE('',*,*,#2792,.F.);
#4103=ORIENTED_EDGE('',*,*,#2992,.F.);
#4104=ORIENTED_EDGE('',*,*,#2871,.F.);
#4105=ORIENTED_EDGE('',*,*,#2993,.F.);
#4106=ORIENTED_EDGE('',*,*,#2864,.T.);
#4107=ORIENTED_EDGE('',*,*,#2994,.T.);
#4108=ORIENTED_EDGE('',*,*,#2799,.F.);
#4109=ORIENTED_EDGE('',*,*,#2660,.F.);
#4110=ORIENTED_EDGE('',*,*,#2802,.F.);
#4111=ORIENTED_EDGE('',*,*,#2549,.T.);
#4112=ORIENTED_EDGE('',*,*,#2861,.T.);
#4113=ORIENTED_EDGE('',*,*,#2652,.F.);
#4114=ORIENTED_EDGE('',*,*,#2862,.T.);
#4115=ORIENTED_EDGE('',*,*,#2551,.T.);
#4116=ORIENTED_EDGE('',*,*,#2801,.F.);
#4117=ORIENTED_EDGE('',*,*,#2995,.T.);
#4118=ORIENTED_EDGE('',*,*,#2800,.F.);
#4119=ORIENTED_EDGE('',*,*,#2994,.F.);
#4120=ORIENTED_EDGE('',*,*,#2863,.F.);
#4121=ORIENTED_EDGE('',*,*,#2995,.F.);
#4122=ORIENTED_EDGE('',*,*,#2868,.T.);
#4123=ORIENTED_EDGE('',*,*,#2996,.T.);
#4124=ORIENTED_EDGE('',*,*,#2795,.F.);
#4125=ORIENTED_EDGE('',*,*,#2654,.F.);
#4126=ORIENTED_EDGE('',*,*,#2798,.F.);
#4127=ORIENTED_EDGE('',*,*,#2545,.T.);
#4128=ORIENTED_EDGE('',*,*,#2865,.T.);
#4129=ORIENTED_EDGE('',*,*,#2658,.F.);
#4130=ORIENTED_EDGE('',*,*,#2866,.T.);
#4131=ORIENTED_EDGE('',*,*,#2547,.T.);
#4132=ORIENTED_EDGE('',*,*,#2797,.F.);
#4133=ORIENTED_EDGE('',*,*,#2997,.T.);
#4134=ORIENTED_EDGE('',*,*,#2796,.F.);
#4135=ORIENTED_EDGE('',*,*,#2996,.F.);
#4136=ORIENTED_EDGE('',*,*,#2867,.F.);
#4137=ORIENTED_EDGE('',*,*,#2997,.F.);
#4138=ORIENTED_EDGE('',*,*,#2860,.T.);
#4139=ORIENTED_EDGE('',*,*,#2998,.T.);
#4140=ORIENTED_EDGE('',*,*,#2803,.F.);
#4141=ORIENTED_EDGE('',*,*,#2650,.F.);
#4142=ORIENTED_EDGE('',*,*,#2858,.T.);
#4143=ORIENTED_EDGE('',*,*,#2540,.T.);
#4144=ORIENTED_EDGE('',*,*,#2805,.F.);
#4145=ORIENTED_EDGE('',*,*,#2999,.T.);
#4146=ORIENTED_EDGE('',*,*,#2804,.F.);
#4147=ORIENTED_EDGE('',*,*,#2998,.F.);
#4148=ORIENTED_EDGE('',*,*,#2859,.F.);
#4149=ORIENTED_EDGE('',*,*,#2999,.F.);
#4150=ORIENTED_EDGE('',*,*,#2857,.T.);
#4151=ORIENTED_EDGE('',*,*,#3000,.T.);
#4152=ORIENTED_EDGE('',*,*,#2806,.F.);
#4153=ORIENTED_EDGE('',*,*,#2647,.F.);
#4154=ORIENTED_EDGE('',*,*,#2855,.T.);
#4155=ORIENTED_EDGE('',*,*,#2533,.T.);
#4156=ORIENTED_EDGE('',*,*,#2808,.F.);
#4157=ORIENTED_EDGE('',*,*,#3001,.T.);
#4158=ORIENTED_EDGE('',*,*,#2807,.F.);
#4159=ORIENTED_EDGE('',*,*,#3000,.F.);
#4160=ORIENTED_EDGE('',*,*,#2856,.F.);
#4161=ORIENTED_EDGE('',*,*,#3001,.F.);
#4162=ORIENTED_EDGE('',*,*,#2762,.F.);
#4163=ORIENTED_EDGE('',*,*,#3002,.T.);
#4164=ORIENTED_EDGE('',*,*,#2901,.T.);
#4165=ORIENTED_EDGE('',*,*,#2682,.F.);
#4166=ORIENTED_EDGE('',*,*,#2761,.F.);
#4167=ORIENTED_EDGE('',*,*,#3003,.F.);
#4168=ORIENTED_EDGE('',*,*,#2902,.F.);
#4169=ORIENTED_EDGE('',*,*,#3002,.F.);
#4170=ORIENTED_EDGE('',*,*,#2903,.T.);
#4171=ORIENTED_EDGE('',*,*,#3003,.T.);
#4172=ORIENTED_EDGE('',*,*,#2760,.F.);
#4173=ORIENTED_EDGE('',*,*,#2524,.T.);
#4174=ORIENTED_EDGE('',*,*,#2759,.F.);
#4175=ORIENTED_EDGE('',*,*,#3004,.T.);
#4176=ORIENTED_EDGE('',*,*,#2904,.T.);
#4177=ORIENTED_EDGE('',*,*,#2644,.F.);
#4178=ORIENTED_EDGE('',*,*,#2758,.F.);
#4179=ORIENTED_EDGE('',*,*,#3005,.F.);
#4180=ORIENTED_EDGE('',*,*,#2905,.F.);
#4181=ORIENTED_EDGE('',*,*,#3004,.F.);
#4182=ORIENTED_EDGE('',*,*,#2906,.T.);
#4183=ORIENTED_EDGE('',*,*,#3005,.T.);
#4184=ORIENTED_EDGE('',*,*,#2757,.F.);
#4185=ORIENTED_EDGE('',*,*,#2517,.T.);
#4186=ORIENTED_EDGE('',*,*,#2911,.T.);
#4187=ORIENTED_EDGE('',*,*,#3006,.T.);
#4188=ORIENTED_EDGE('',*,*,#2752,.F.);
#4189=ORIENTED_EDGE('',*,*,#2639,.F.);
#4190=ORIENTED_EDGE('',*,*,#2756,.F.);
#4191=ORIENTED_EDGE('',*,*,#3007,.T.);
#4192=ORIENTED_EDGE('',*,*,#2907,.T.);
#4193=ORIENTED_EDGE('',*,*,#2641,.F.);
#4194=ORIENTED_EDGE('',*,*,#2755,.F.);
#4195=ORIENTED_EDGE('',*,*,#3008,.F.);
#4196=ORIENTED_EDGE('',*,*,#2908,.F.);
#4197=ORIENTED_EDGE('',*,*,#3007,.F.);
#4198=ORIENTED_EDGE('',*,*,#2909,.T.);
#4199=ORIENTED_EDGE('',*,*,#3008,.T.);
#4200=ORIENTED_EDGE('',*,*,#2754,.F.);
#4201=ORIENTED_EDGE('',*,*,#3009,.T.);
#4202=ORIENTED_EDGE('',*,*,#2753,.F.);
#4203=ORIENTED_EDGE('',*,*,#3006,.F.);
#4204=ORIENTED_EDGE('',*,*,#2910,.F.);
#4205=ORIENTED_EDGE('',*,*,#3009,.F.);
#4206=ORIENTED_EDGE('',*,*,#2916,.T.);
#4207=ORIENTED_EDGE('',*,*,#3010,.T.);
#4208=ORIENTED_EDGE('',*,*,#2747,.F.);
#4209=ORIENTED_EDGE('',*,*,#2635,.F.);
#4210=ORIENTED_EDGE('',*,*,#2751,.F.);
#4211=ORIENTED_EDGE('',*,*,#3011,.T.);
#4212=ORIENTED_EDGE('',*,*,#2912,.T.);
#4213=ORIENTED_EDGE('',*,*,#2637,.F.);
#4214=ORIENTED_EDGE('',*,*,#2750,.F.);
#4215=ORIENTED_EDGE('',*,*,#3012,.F.);
#4216=ORIENTED_EDGE('',*,*,#2913,.F.);
#4217=ORIENTED_EDGE('',*,*,#3011,.F.);
#4218=ORIENTED_EDGE('',*,*,#2914,.T.);
#4219=ORIENTED_EDGE('',*,*,#3012,.T.);
#4220=ORIENTED_EDGE('',*,*,#2749,.F.);
#4221=ORIENTED_EDGE('',*,*,#3013,.T.);
#4222=ORIENTED_EDGE('',*,*,#2748,.F.);
#4223=ORIENTED_EDGE('',*,*,#3010,.F.);
#4224=ORIENTED_EDGE('',*,*,#2915,.F.);
#4225=ORIENTED_EDGE('',*,*,#3013,.F.);
#4226=ORIENTED_EDGE('',*,*,#2931,.T.);
#4227=ORIENTED_EDGE('',*,*,#3014,.T.);
#4228=ORIENTED_EDGE('',*,*,#2732,.F.);
#4229=ORIENTED_EDGE('',*,*,#2631,.F.);
#4230=ORIENTED_EDGE('',*,*,#2736,.F.);
#4231=ORIENTED_EDGE('',*,*,#3015,.T.);
#4232=ORIENTED_EDGE('',*,*,#2927,.T.);
#4233=ORIENTED_EDGE('',*,*,#2623,.F.);
#4234=ORIENTED_EDGE('',*,*,#2735,.F.);
#4235=ORIENTED_EDGE('',*,*,#3016,.F.);
#4236=ORIENTED_EDGE('',*,*,#2928,.F.);
#4237=ORIENTED_EDGE('',*,*,#3015,.F.);
#4238=ORIENTED_EDGE('',*,*,#2929,.T.);
#4239=ORIENTED_EDGE('',*,*,#3016,.T.);
#4240=ORIENTED_EDGE('',*,*,#2734,.F.);
#4241=ORIENTED_EDGE('',*,*,#3017,.T.);
#4242=ORIENTED_EDGE('',*,*,#2733,.F.);
#4243=ORIENTED_EDGE('',*,*,#3014,.F.);
#4244=ORIENTED_EDGE('',*,*,#2930,.F.);
#4245=ORIENTED_EDGE('',*,*,#3017,.F.);
#4246=ORIENTED_EDGE('',*,*,#2936,.T.);
#4247=ORIENTED_EDGE('',*,*,#3018,.T.);
#4248=ORIENTED_EDGE('',*,*,#2727,.F.);
#4249=ORIENTED_EDGE('',*,*,#2627,.F.);
#4250=ORIENTED_EDGE('',*,*,#2731,.F.);
#4251=ORIENTED_EDGE('',*,*,#3019,.T.);
#4252=ORIENTED_EDGE('',*,*,#2932,.T.);
#4253=ORIENTED_EDGE('',*,*,#2629,.F.);
#4254=ORIENTED_EDGE('',*,*,#2730,.F.);
#4255=ORIENTED_EDGE('',*,*,#3020,.F.);
#4256=ORIENTED_EDGE('',*,*,#2933,.F.);
#4257=ORIENTED_EDGE('',*,*,#3019,.F.);
#4258=ORIENTED_EDGE('',*,*,#2934,.T.);
#4259=ORIENTED_EDGE('',*,*,#3020,.T.);
#4260=ORIENTED_EDGE('',*,*,#2729,.F.);
#4261=ORIENTED_EDGE('',*,*,#3021,.T.);
#4262=ORIENTED_EDGE('',*,*,#2728,.F.);
#4263=ORIENTED_EDGE('',*,*,#3018,.F.);
#4264=ORIENTED_EDGE('',*,*,#2935,.F.);
#4265=ORIENTED_EDGE('',*,*,#3021,.F.);
#4266=ORIENTED_EDGE('',*,*,#2926,.T.);
#4267=ORIENTED_EDGE('',*,*,#3022,.T.);
#4268=ORIENTED_EDGE('',*,*,#2737,.F.);
#4269=ORIENTED_EDGE('',*,*,#2621,.F.);
#4270=ORIENTED_EDGE('',*,*,#2741,.F.);
#4271=ORIENTED_EDGE('',*,*,#3023,.T.);
#4272=ORIENTED_EDGE('',*,*,#2922,.T.);
#4273=ORIENTED_EDGE('',*,*,#2619,.F.);
#4274=ORIENTED_EDGE('',*,*,#2740,.F.);
#4275=ORIENTED_EDGE('',*,*,#3024,.F.);
#4276=ORIENTED_EDGE('',*,*,#2923,.F.);
#4277=ORIENTED_EDGE('',*,*,#3023,.F.);
#4278=ORIENTED_EDGE('',*,*,#2924,.T.);
#4279=ORIENTED_EDGE('',*,*,#3024,.T.);
#4280=ORIENTED_EDGE('',*,*,#2739,.F.);
#4281=ORIENTED_EDGE('',*,*,#3025,.T.);
#4282=ORIENTED_EDGE('',*,*,#2738,.F.);
#4283=ORIENTED_EDGE('',*,*,#3022,.F.);
#4284=ORIENTED_EDGE('',*,*,#2925,.F.);
#4285=ORIENTED_EDGE('',*,*,#3025,.F.);
#4286=ORIENTED_EDGE('',*,*,#2921,.T.);
#4287=ORIENTED_EDGE('',*,*,#3026,.T.);
#4288=ORIENTED_EDGE('',*,*,#2742,.F.);
#4289=ORIENTED_EDGE('',*,*,#2617,.F.);
#4290=ORIENTED_EDGE('',*,*,#2746,.F.);
#4291=ORIENTED_EDGE('',*,*,#3027,.T.);
#4292=ORIENTED_EDGE('',*,*,#2917,.T.);
#4293=ORIENTED_EDGE('',*,*,#2633,.F.);
#4294=ORIENTED_EDGE('',*,*,#2745,.F.);
#4295=ORIENTED_EDGE('',*,*,#3028,.F.);
#4296=ORIENTED_EDGE('',*,*,#2918,.F.);
#4297=ORIENTED_EDGE('',*,*,#3027,.F.);
#4298=ORIENTED_EDGE('',*,*,#2919,.T.);
#4299=ORIENTED_EDGE('',*,*,#3028,.T.);
#4300=ORIENTED_EDGE('',*,*,#2744,.F.);
#4301=ORIENTED_EDGE('',*,*,#3029,.T.);
#4302=ORIENTED_EDGE('',*,*,#2743,.F.);
#4303=ORIENTED_EDGE('',*,*,#3026,.F.);
#4304=ORIENTED_EDGE('',*,*,#2920,.F.);
#4305=ORIENTED_EDGE('',*,*,#3029,.F.);
#4306=ORIENTED_EDGE('',*,*,#2941,.T.);
#4307=ORIENTED_EDGE('',*,*,#3030,.T.);
#4308=ORIENTED_EDGE('',*,*,#2722,.F.);
#4309=ORIENTED_EDGE('',*,*,#2615,.F.);
#4310=ORIENTED_EDGE('',*,*,#2726,.F.);
#4311=ORIENTED_EDGE('',*,*,#3031,.T.);
#4312=ORIENTED_EDGE('',*,*,#2937,.T.);
#4313=ORIENTED_EDGE('',*,*,#2625,.F.);
#4314=ORIENTED_EDGE('',*,*,#2725,.F.);
#4315=ORIENTED_EDGE('',*,*,#3032,.F.);
#4316=ORIENTED_EDGE('',*,*,#2938,.F.);
#4317=ORIENTED_EDGE('',*,*,#3031,.F.);
#4318=ORIENTED_EDGE('',*,*,#2939,.T.);
#4319=ORIENTED_EDGE('',*,*,#3032,.T.);
#4320=ORIENTED_EDGE('',*,*,#2724,.F.);
#4321=ORIENTED_EDGE('',*,*,#3033,.T.);
#4322=ORIENTED_EDGE('',*,*,#2723,.F.);
#4323=ORIENTED_EDGE('',*,*,#3030,.F.);
#4324=ORIENTED_EDGE('',*,*,#2940,.F.);
#4325=ORIENTED_EDGE('',*,*,#3033,.F.);
#4326=ORIENTED_EDGE('',*,*,#2946,.T.);
#4327=ORIENTED_EDGE('',*,*,#3034,.T.);
#4328=ORIENTED_EDGE('',*,*,#2717,.F.);
#4329=ORIENTED_EDGE('',*,*,#2585,.F.);
#4330=ORIENTED_EDGE('',*,*,#2721,.F.);
#4331=ORIENTED_EDGE('',*,*,#3035,.T.);
#4332=ORIENTED_EDGE('',*,*,#2942,.T.);
#4333=ORIENTED_EDGE('',*,*,#2613,.F.);
#4334=ORIENTED_EDGE('',*,*,#2720,.F.);
#4335=ORIENTED_EDGE('',*,*,#3036,.F.);
#4336=ORIENTED_EDGE('',*,*,#2943,.F.);
#4337=ORIENTED_EDGE('',*,*,#3035,.F.);
#4338=ORIENTED_EDGE('',*,*,#2944,.T.);
#4339=ORIENTED_EDGE('',*,*,#3036,.T.);
#4340=ORIENTED_EDGE('',*,*,#2719,.F.);
#4341=ORIENTED_EDGE('',*,*,#3037,.T.);
#4342=ORIENTED_EDGE('',*,*,#2718,.F.);
#4343=ORIENTED_EDGE('',*,*,#3034,.F.);
#4344=ORIENTED_EDGE('',*,*,#2945,.F.);
#4345=ORIENTED_EDGE('',*,*,#3037,.F.);
#4346=ORIENTED_EDGE('',*,*,#2951,.T.);
#4347=ORIENTED_EDGE('',*,*,#3038,.T.);
#4348=ORIENTED_EDGE('',*,*,#2712,.F.);
#4349=ORIENTED_EDGE('',*,*,#2611,.F.);
#4350=ORIENTED_EDGE('',*,*,#2716,.F.);
#4351=ORIENTED_EDGE('',*,*,#3039,.T.);
#4352=ORIENTED_EDGE('',*,*,#2947,.T.);
#4353=ORIENTED_EDGE('',*,*,#2587,.F.);
#4354=ORIENTED_EDGE('',*,*,#2715,.F.);
#4355=ORIENTED_EDGE('',*,*,#3040,.F.);
#4356=ORIENTED_EDGE('',*,*,#2948,.F.);
#4357=ORIENTED_EDGE('',*,*,#3039,.F.);
#4358=ORIENTED_EDGE('',*,*,#2949,.T.);
#4359=ORIENTED_EDGE('',*,*,#3040,.T.);
#4360=ORIENTED_EDGE('',*,*,#2714,.F.);
#4361=ORIENTED_EDGE('',*,*,#3041,.T.);
#4362=ORIENTED_EDGE('',*,*,#2713,.F.);
#4363=ORIENTED_EDGE('',*,*,#3038,.F.);
#4364=ORIENTED_EDGE('',*,*,#2950,.F.);
#4365=ORIENTED_EDGE('',*,*,#3041,.F.);
#4366=ORIENTED_EDGE('',*,*,#2956,.T.);
#4367=ORIENTED_EDGE('',*,*,#3042,.T.);
#4368=ORIENTED_EDGE('',*,*,#2707,.F.);
#4369=ORIENTED_EDGE('',*,*,#2607,.F.);
#4370=ORIENTED_EDGE('',*,*,#2711,.F.);
#4371=ORIENTED_EDGE('',*,*,#3043,.T.);
#4372=ORIENTED_EDGE('',*,*,#2952,.T.);
#4373=ORIENTED_EDGE('',*,*,#2609,.F.);
#4374=ORIENTED_EDGE('',*,*,#2710,.F.);
#4375=ORIENTED_EDGE('',*,*,#3044,.F.);
#4376=ORIENTED_EDGE('',*,*,#2953,.F.);
#4377=ORIENTED_EDGE('',*,*,#3043,.F.);
#4378=ORIENTED_EDGE('',*,*,#2954,.T.);
#4379=ORIENTED_EDGE('',*,*,#3044,.T.);
#4380=ORIENTED_EDGE('',*,*,#2709,.F.);
#4381=ORIENTED_EDGE('',*,*,#3045,.T.);
#4382=ORIENTED_EDGE('',*,*,#2708,.F.);
#4383=ORIENTED_EDGE('',*,*,#3042,.F.);
#4384=ORIENTED_EDGE('',*,*,#2955,.F.);
#4385=ORIENTED_EDGE('',*,*,#3045,.F.);
#4386=ORIENTED_EDGE('',*,*,#2843,.T.);
#4387=ORIENTED_EDGE('',*,*,#3046,.T.);
#4388=ORIENTED_EDGE('',*,*,#2820,.F.);
#4389=ORIENTED_EDGE('',*,*,#2601,.F.);
#4390=ORIENTED_EDGE('',*,*,#2824,.F.);
#4391=ORIENTED_EDGE('',*,*,#3047,.T.);
#4392=ORIENTED_EDGE('',*,*,#2839,.T.);
#4393=ORIENTED_EDGE('',*,*,#2599,.F.);
#4394=ORIENTED_EDGE('',*,*,#2823,.F.);
#4395=ORIENTED_EDGE('',*,*,#3048,.F.);
#4396=ORIENTED_EDGE('',*,*,#2840,.F.);
#4397=ORIENTED_EDGE('',*,*,#3047,.F.);
#4398=ORIENTED_EDGE('',*,*,#2841,.T.);
#4399=ORIENTED_EDGE('',*,*,#3048,.T.);
#4400=ORIENTED_EDGE('',*,*,#2822,.F.);
#4401=ORIENTED_EDGE('',*,*,#3049,.T.);
#4402=ORIENTED_EDGE('',*,*,#2821,.F.);
#4403=ORIENTED_EDGE('',*,*,#3046,.F.);
#4404=ORIENTED_EDGE('',*,*,#2842,.F.);
#4405=ORIENTED_EDGE('',*,*,#3049,.F.);
#4406=ORIENTED_EDGE('',*,*,#2838,.T.);
#4407=ORIENTED_EDGE('',*,*,#3050,.T.);
#4408=ORIENTED_EDGE('',*,*,#2825,.F.);
#4409=ORIENTED_EDGE('',*,*,#2597,.F.);
#4410=ORIENTED_EDGE('',*,*,#2829,.F.);
#4411=ORIENTED_EDGE('',*,*,#3051,.T.);
#4412=ORIENTED_EDGE('',*,*,#2834,.T.);
#4413=ORIENTED_EDGE('',*,*,#2591,.F.);
#4414=ORIENTED_EDGE('',*,*,#2828,.F.);
#4415=ORIENTED_EDGE('',*,*,#3052,.F.);
#4416=ORIENTED_EDGE('',*,*,#2835,.F.);
#4417=ORIENTED_EDGE('',*,*,#3051,.F.);
#4418=ORIENTED_EDGE('',*,*,#2836,.T.);
#4419=ORIENTED_EDGE('',*,*,#3052,.T.);
#4420=ORIENTED_EDGE('',*,*,#2827,.F.);
#4421=ORIENTED_EDGE('',*,*,#3053,.T.);
#4422=ORIENTED_EDGE('',*,*,#2826,.F.);
#4423=ORIENTED_EDGE('',*,*,#3050,.F.);
#4424=ORIENTED_EDGE('',*,*,#2837,.F.);
#4425=ORIENTED_EDGE('',*,*,#3053,.F.);
#4426=ORIENTED_EDGE('',*,*,#2961,.T.);
#4427=ORIENTED_EDGE('',*,*,#3054,.T.);
#4428=ORIENTED_EDGE('',*,*,#2702,.F.);
#4429=ORIENTED_EDGE('',*,*,#2595,.F.);
#4430=ORIENTED_EDGE('',*,*,#2706,.F.);
#4431=ORIENTED_EDGE('',*,*,#3055,.T.);
#4432=ORIENTED_EDGE('',*,*,#2957,.T.);
#4433=ORIENTED_EDGE('',*,*,#2605,.F.);
#4434=ORIENTED_EDGE('',*,*,#2705,.F.);
#4435=ORIENTED_EDGE('',*,*,#3056,.F.);
#4436=ORIENTED_EDGE('',*,*,#2958,.F.);
#4437=ORIENTED_EDGE('',*,*,#3055,.F.);
#4438=ORIENTED_EDGE('',*,*,#2959,.T.);
#4439=ORIENTED_EDGE('',*,*,#3056,.T.);
#4440=ORIENTED_EDGE('',*,*,#2704,.F.);
#4441=ORIENTED_EDGE('',*,*,#3057,.T.);
#4442=ORIENTED_EDGE('',*,*,#2703,.F.);
#4443=ORIENTED_EDGE('',*,*,#3054,.F.);
#4444=ORIENTED_EDGE('',*,*,#2960,.F.);
#4445=ORIENTED_EDGE('',*,*,#3057,.F.);
#4446=ORIENTED_EDGE('',*,*,#2833,.T.);
#4447=ORIENTED_EDGE('',*,*,#3058,.T.);
#4448=ORIENTED_EDGE('',*,*,#2697,.F.);
#4449=ORIENTED_EDGE('',*,*,#2589,.F.);
#4450=ORIENTED_EDGE('',*,*,#2701,.F.);
#4451=ORIENTED_EDGE('',*,*,#3059,.T.);
#4452=ORIENTED_EDGE('',*,*,#2962,.T.);
#4453=ORIENTED_EDGE('',*,*,#2593,.F.);
#4454=ORIENTED_EDGE('',*,*,#2700,.F.);
#4455=ORIENTED_EDGE('',*,*,#3060,.F.);
#4456=ORIENTED_EDGE('',*,*,#2963,.F.);
#4457=ORIENTED_EDGE('',*,*,#3059,.F.);
#4458=ORIENTED_EDGE('',*,*,#2964,.T.);
#4459=ORIENTED_EDGE('',*,*,#3060,.T.);
#4460=ORIENTED_EDGE('',*,*,#2699,.F.);
#4461=ORIENTED_EDGE('',*,*,#3061,.T.);
#4462=ORIENTED_EDGE('',*,*,#2698,.F.);
#4463=ORIENTED_EDGE('',*,*,#3058,.F.);
#4464=ORIENTED_EDGE('',*,*,#2965,.F.);
#4465=ORIENTED_EDGE('',*,*,#3061,.F.);
#4466=ORIENTED_EDGE('',*,*,#3062,.T.);
#4467=ORIENTED_EDGE('',*,*,#2967,.T.);
#4468=ORIENTED_EDGE('',*,*,#3063,.F.);
#4469=ORIENTED_EDGE('',*,*,#2830,.F.);
#4470=ORIENTED_EDGE('',*,*,#3063,.T.);
#4471=ORIENTED_EDGE('',*,*,#2966,.T.);
#4472=ORIENTED_EDGE('',*,*,#2513,.F.);
#4473=ORIENTED_EDGE('',*,*,#2831,.F.);
#4474=ORIENTED_EDGE('',*,*,#2515,.F.);
#4475=ORIENTED_EDGE('',*,*,#2968,.T.);
#4476=ORIENTED_EDGE('',*,*,#3062,.F.);
#4477=ORIENTED_EDGE('',*,*,#2832,.F.);
#4808=CYLINDRICAL_SURFACE('',#5467,4.5);
#4809=CYLINDRICAL_SURFACE('',#5470,0.405000000000001);
#4810=CYLINDRICAL_SURFACE('',#5473,5.53127226019911);
#4811=CYLINDRICAL_SURFACE('',#5476,0.404999999999999);
#4812=CYLINDRICAL_SURFACE('',#5479,5.53127226019911);
#4813=CYLINDRICAL_SURFACE('',#5482,0.405);
#4814=CYLINDRICAL_SURFACE('',#5485,5.53127226019911);
#4815=CYLINDRICAL_SURFACE('',#5488,0.404999999999999);
#4816=CYLINDRICAL_SURFACE('',#5491,5.53127226019911);
#4817=CYLINDRICAL_SURFACE('',#5494,0.404999999999999);
#4818=CYLINDRICAL_SURFACE('',#5497,0.404999999999999);
#4819=CYLINDRICAL_SURFACE('',#5500,0.404999999999999);
#4820=CYLINDRICAL_SURFACE('',#5503,0.404999999999999);
#4821=CYLINDRICAL_SURFACE('',#5506,0.404999999999999);
#4822=CYLINDRICAL_SURFACE('',#5509,0.404999999999999);
#4823=CYLINDRICAL_SURFACE('',#5512,0.404999999999999);
#4824=CYLINDRICAL_SURFACE('',#5515,0.404999999999999);
#4825=CYLINDRICAL_SURFACE('',#5518,0.404999999999999);
#4826=CYLINDRICAL_SURFACE('',#5521,0.404999999999999);
#4827=CYLINDRICAL_SURFACE('',#5524,21.6);
#4828=CYLINDRICAL_SURFACE('',#5527,21.6);
#4829=CYLINDRICAL_SURFACE('',#5530,21.6);
#4830=CYLINDRICAL_SURFACE('',#5533,21.6);
#4831=CYLINDRICAL_SURFACE('',#5536,21.6);
#4832=CYLINDRICAL_SURFACE('',#5539,21.6);
#4833=CYLINDRICAL_SURFACE('',#5542,21.6);
#4834=CYLINDRICAL_SURFACE('',#5545,21.6);
#4835=CYLINDRICAL_SURFACE('',#5548,21.6);
#4836=CYLINDRICAL_SURFACE('',#5551,21.6);
#4837=CYLINDRICAL_SURFACE('',#5554,21.6);
#4838=CYLINDRICAL_SURFACE('',#5557,21.6);
#4839=CYLINDRICAL_SURFACE('',#5560,21.6);
#4840=CYLINDRICAL_SURFACE('',#5563,21.6);
#4841=CYLINDRICAL_SURFACE('',#5566,21.6);
#4842=CYLINDRICAL_SURFACE('',#5569,21.6);
#4843=CYLINDRICAL_SURFACE('',#5572,21.6);
#4844=CYLINDRICAL_SURFACE('',#5575,21.6);
#4845=CYLINDRICAL_SURFACE('',#5578,21.6);
#4846=CYLINDRICAL_SURFACE('',#5581,21.6);
#4847=CYLINDRICAL_SURFACE('',#5584,21.6);
#4848=CYLINDRICAL_SURFACE('',#5587,21.6);
#4849=CYLINDRICAL_SURFACE('',#5590,21.6);
#4850=CYLINDRICAL_SURFACE('',#5593,21.6);
#4851=CYLINDRICAL_SURFACE('',#5596,21.6);
#4852=CYLINDRICAL_SURFACE('',#5599,21.6);
#4853=CYLINDRICAL_SURFACE('',#5602,21.6);
#4854=CYLINDRICAL_SURFACE('',#5605,21.6);
#4855=CYLINDRICAL_SURFACE('',#5608,21.6);
#4856=CYLINDRICAL_SURFACE('',#5879,21.6);
#4857=CYLINDRICAL_SURFACE('',#5880,5.53127226019911);
#4858=CYLINDRICAL_SURFACE('',#5881,5.53127226019911);
#4859=CYLINDRICAL_SURFACE('',#5882,18.5625);
#4860=CYLINDRICAL_SURFACE('',#5883,0.405);
#4861=CYLINDRICAL_SURFACE('',#5884,0.405);
#4862=CYLINDRICAL_SURFACE('',#5885,5.53127226019911);
#4863=CYLINDRICAL_SURFACE('',#5886,5.53127226019911);
#4864=CYLINDRICAL_SURFACE('',#5887,0.405);
#4865=CYLINDRICAL_SURFACE('',#5888,18.5625);
#4866=CYLINDRICAL_SURFACE('',#5889,0.405000000000001);
#4867=CYLINDRICAL_SURFACE('',#5890,5.53127226019911);
#4868=CYLINDRICAL_SURFACE('',#5891,5.53127226019911);
#4869=CYLINDRICAL_SURFACE('',#5892,0.404999999999999);
#4870=CYLINDRICAL_SURFACE('',#5893,18.5625);
#4871=CYLINDRICAL_SURFACE('',#5894,5.53127226019911);
#4872=CYLINDRICAL_SURFACE('',#5895,5.53127226019911);
#4873=CYLINDRICAL_SURFACE('',#5896,0.404999999999999);
#4874=CYLINDRICAL_SURFACE('',#5897,18.5625);
#4875=CYLINDRICAL_SURFACE('',#5898,5.53127226019911);
#4876=CYLINDRICAL_SURFACE('',#5899,5.53127226019911);
#4877=CYLINDRICAL_SURFACE('',#5900,0.404999999999999);
#4878=CYLINDRICAL_SURFACE('',#5901,18.5625);
#4879=CYLINDRICAL_SURFACE('',#5902,5.53127226019911);
#4880=CYLINDRICAL_SURFACE('',#5903,5.53127226019911);
#4881=CYLINDRICAL_SURFACE('',#5904,0.404999999999999);
#4882=CYLINDRICAL_SURFACE('',#5905,18.5625);
#4883=CYLINDRICAL_SURFACE('',#5906,5.53127226019911);
#4884=CYLINDRICAL_SURFACE('',#5907,5.53127226019911);
#4885=CYLINDRICAL_SURFACE('',#5908,0.404999999999999);
#4886=CYLINDRICAL_SURFACE('',#5909,18.5625);
#4887=CYLINDRICAL_SURFACE('',#5910,5.53127226019911);
#4888=CYLINDRICAL_SURFACE('',#5911,5.53127226019911);
#4889=CYLINDRICAL_SURFACE('',#5912,18.5625);
#4890=CYLINDRICAL_SURFACE('',#5913,0.404999999999999);
#4891=CYLINDRICAL_SURFACE('',#5914,5.53127226019911);
#4892=CYLINDRICAL_SURFACE('',#5915,5.53127226019911);
#4893=CYLINDRICAL_SURFACE('',#5916,18.5625);
#4894=CYLINDRICAL_SURFACE('',#5917,0.404999999999999);
#4895=CYLINDRICAL_SURFACE('',#5918,5.53127226019911);
#4896=CYLINDRICAL_SURFACE('',#5919,5.53127226019911);
#4897=CYLINDRICAL_SURFACE('',#5920,18.5625);
#4898=CYLINDRICAL_SURFACE('',#5921,0.404999999999999);
#4899=CYLINDRICAL_SURFACE('',#5922,5.53127226019911);
#4900=CYLINDRICAL_SURFACE('',#5923,5.53127226019911);
#4901=CYLINDRICAL_SURFACE('',#5924,18.5625);
#4902=CYLINDRICAL_SURFACE('',#5925,0.404999999999999);
#4903=CYLINDRICAL_SURFACE('',#5926,5.53127226019911);
#4904=CYLINDRICAL_SURFACE('',#5927,5.53127226019911);
#4905=CYLINDRICAL_SURFACE('',#5928,18.5625);
#4906=CYLINDRICAL_SURFACE('',#5929,0.404999999999999);
#4907=CYLINDRICAL_SURFACE('',#5930,5.53127226019911);
#4908=CYLINDRICAL_SURFACE('',#5931,18.5625);
#4909=CYLINDRICAL_SURFACE('',#5932,0.404999999999999);
#4910=CYLINDRICAL_SURFACE('',#5933,5.53127226019911);
#4911=CYLINDRICAL_SURFACE('',#5934,18.5625);
#4912=CYLINDRICAL_SURFACE('',#5935,0.405000000000001);
#4913=CYLINDRICAL_SURFACE('',#5936,5.53127226019911);
#4914=CYLINDRICAL_SURFACE('',#5937,0.405000000000001);
#4915=CYLINDRICAL_SURFACE('',#5938,18.5625);
#4916=CYLINDRICAL_SURFACE('',#5939,5.53127226019911);
#4917=CYLINDRICAL_SURFACE('',#5940,0.405);
#4918=CYLINDRICAL_SURFACE('',#5941,18.5625);
#4919=CYLINDRICAL_SURFACE('',#5942,5.53127226019911);
#4920=CYLINDRICAL_SURFACE('',#5943,5.53127226019911);
#4921=CYLINDRICAL_SURFACE('',#5944,0.405);
#4922=CYLINDRICAL_SURFACE('',#5945,18.5625);
#4923=CYLINDRICAL_SURFACE('',#5946,0.405);
#4924=CYLINDRICAL_SURFACE('',#5947,5.53127226019911);
#4925=CYLINDRICAL_SURFACE('',#5948,5.53127226019911);
#4926=CYLINDRICAL_SURFACE('',#5949,0.405);
#4927=CYLINDRICAL_SURFACE('',#5950,18.5625);
#4928=CYLINDRICAL_SURFACE('',#5951,0.404999999999999);
#4929=CYLINDRICAL_SURFACE('',#5952,5.53127226019911);
#4930=CYLINDRICAL_SURFACE('',#5953,5.53127226019911);
#4931=CYLINDRICAL_SURFACE('',#5954,0.404999999999999);
#4932=CYLINDRICAL_SURFACE('',#5955,18.5625);
#4933=CYLINDRICAL_SURFACE('',#5956,0.404999999999999);
#4934=CYLINDRICAL_SURFACE('',#5957,5.53127226019911);
#4935=CYLINDRICAL_SURFACE('',#5958,5.53127226019911);
#4936=CYLINDRICAL_SURFACE('',#5959,0.404999999999999);
#4937=CYLINDRICAL_SURFACE('',#5960,18.5625);
#4938=CYLINDRICAL_SURFACE('',#5961,0.404999999999999);
#4939=CYLINDRICAL_SURFACE('',#5962,5.53127226019911);
#4940=CYLINDRICAL_SURFACE('',#5963,5.53127226019911);
#4941=CYLINDRICAL_SURFACE('',#5964,0.404999999999999);
#4942=CYLINDRICAL_SURFACE('',#5965,18.5625);
#4943=CYLINDRICAL_SURFACE('',#5966,0.404999999999999);
#4944=CYLINDRICAL_SURFACE('',#5967,5.53127226019911);
#4945=CYLINDRICAL_SURFACE('',#5968,5.53127226019911);
#4946=CYLINDRICAL_SURFACE('',#5969,0.405000000000001);
#4947=CYLINDRICAL_SURFACE('',#5970,18.5625);
#4948=CYLINDRICAL_SURFACE('',#5971,0.404999999999999);
#4949=CYLINDRICAL_SURFACE('',#5972,5.53127226019911);
#4950=CYLINDRICAL_SURFACE('',#5973,5.53127226019911);
#4951=CYLINDRICAL_SURFACE('',#5974,0.404999999999999);
#4952=CYLINDRICAL_SURFACE('',#5975,18.5625);
#4953=CYLINDRICAL_SURFACE('',#5976,0.404999999999999);
#4954=CYLINDRICAL_SURFACE('',#5977,5.53127226019911);
#4955=CYLINDRICAL_SURFACE('',#5978,5.53127226019911);
#4956=CYLINDRICAL_SURFACE('',#5979,0.404999999999999);
#4957=CYLINDRICAL_SURFACE('',#5980,18.5625);
#4958=CYLINDRICAL_SURFACE('',#5981,0.404999999999999);
#4959=CYLINDRICAL_SURFACE('',#5982,5.53127226019912);
#4960=CYLINDRICAL_SURFACE('',#5983,5.53127226019911);
#4961=CYLINDRICAL_SURFACE('',#5984,0.404999999999999);
#4962=CYLINDRICAL_SURFACE('',#5985,18.5625);
#4963=CYLINDRICAL_SURFACE('',#5986,0.404999999999999);
#4964=CYLINDRICAL_SURFACE('',#5987,5.53127226019911);
#4965=CYLINDRICAL_SURFACE('',#5988,5.53127226019911);
#4966=CYLINDRICAL_SURFACE('',#5989,0.404999999999999);
#4967=CYLINDRICAL_SURFACE('',#5990,18.5625);
#4968=CYLINDRICAL_SURFACE('',#5991,0.404999999999999);
#4969=CYLINDRICAL_SURFACE('',#5992,5.53127226019911);
#4970=CYLINDRICAL_SURFACE('',#5993,5.53127226019911);
#4971=CYLINDRICAL_SURFACE('',#5994,0.404999999999999);
#4972=CYLINDRICAL_SURFACE('',#5995,18.5625);
#4973=CYLINDRICAL_SURFACE('',#5996,0.404999999999999);
#4974=CYLINDRICAL_SURFACE('',#5997,5.53127226019911);
#4975=CYLINDRICAL_SURFACE('',#5998,5.53127226019911);
#4976=CYLINDRICAL_SURFACE('',#5999,0.404999999999999);
#4977=CYLINDRICAL_SURFACE('',#6000,18.5625);
#4978=CYLINDRICAL_SURFACE('',#6001,0.404999999999999);
#4979=CYLINDRICAL_SURFACE('',#6002,5.53127226019911);
#4980=CYLINDRICAL_SURFACE('',#6003,5.53127226019911);
#4981=CYLINDRICAL_SURFACE('',#6004,0.404999999999999);
#4982=CYLINDRICAL_SURFACE('',#6005,18.5625);
#4983=CYLINDRICAL_SURFACE('',#6006,0.404999999999999);
#4984=CYLINDRICAL_SURFACE('',#6007,5.53127226019911);
#4985=CYLINDRICAL_SURFACE('',#6008,5.53127226019911);
#4986=CYLINDRICAL_SURFACE('',#6009,0.404999999999999);
#4987=CYLINDRICAL_SURFACE('',#6010,18.5625);
#4988=CYLINDRICAL_SURFACE('',#6011,0.404999999999999);
#5044=ADVANCED_FACE('',(#310),#4808,.F.);
#5045=ADVANCED_FACE('',(#311),#4809,.F.);
#5046=ADVANCED_FACE('',(#312),#4810,.T.);
#5047=ADVANCED_FACE('',(#313),#4811,.F.);
#5048=ADVANCED_FACE('',(#314),#4812,.T.);
#5049=ADVANCED_FACE('',(#315),#4813,.F.);
#5050=ADVANCED_FACE('',(#316),#4814,.T.);
#5051=ADVANCED_FACE('',(#317),#4815,.F.);
#5052=ADVANCED_FACE('',(#318),#4816,.T.);
#5053=ADVANCED_FACE('',(#319),#4817,.F.);
#5054=ADVANCED_FACE('',(#320),#4818,.F.);
#5055=ADVANCED_FACE('',(#321),#4819,.F.);
#5056=ADVANCED_FACE('',(#322),#4820,.F.);
#5057=ADVANCED_FACE('',(#323),#4821,.F.);
#5058=ADVANCED_FACE('',(#324),#4822,.F.);
#5059=ADVANCED_FACE('',(#325),#4823,.F.);
#5060=ADVANCED_FACE('',(#326),#4824,.F.);
#5061=ADVANCED_FACE('',(#327),#4825,.F.);
#5062=ADVANCED_FACE('',(#328),#4826,.F.);
#5063=ADVANCED_FACE('',(#329),#4827,.T.);
#5064=ADVANCED_FACE('',(#330),#4828,.T.);
#5065=ADVANCED_FACE('',(#331),#4829,.T.);
#5066=ADVANCED_FACE('',(#332),#4830,.T.);
#5067=ADVANCED_FACE('',(#333),#4831,.T.);
#5068=ADVANCED_FACE('',(#334),#4832,.T.);
#5069=ADVANCED_FACE('',(#335),#4833,.T.);
#5070=ADVANCED_FACE('',(#336),#4834,.T.);
#5071=ADVANCED_FACE('',(#337),#4835,.T.);
#5072=ADVANCED_FACE('',(#338),#4836,.T.);
#5073=ADVANCED_FACE('',(#339),#4837,.T.);
#5074=ADVANCED_FACE('',(#340),#4838,.T.);
#5075=ADVANCED_FACE('',(#341),#4839,.T.);
#5076=ADVANCED_FACE('',(#342),#4840,.T.);
#5077=ADVANCED_FACE('',(#343),#4841,.T.);
#5078=ADVANCED_FACE('',(#344),#4842,.T.);
#5079=ADVANCED_FACE('',(#345),#4843,.T.);
#5080=ADVANCED_FACE('',(#346),#4844,.T.);
#5081=ADVANCED_FACE('',(#347),#4845,.T.);
#5082=ADVANCED_FACE('',(#348),#4846,.T.);
#5083=ADVANCED_FACE('',(#349),#4847,.T.);
#5084=ADVANCED_FACE('',(#350),#4848,.T.);
#5085=ADVANCED_FACE('',(#351),#4849,.T.);
#5086=ADVANCED_FACE('',(#352),#4850,.T.);
#5087=ADVANCED_FACE('',(#353),#4851,.T.);
#5088=ADVANCED_FACE('',(#354),#4852,.T.);
#5089=ADVANCED_FACE('',(#355),#4853,.T.);
#5090=ADVANCED_FACE('',(#356),#4854,.T.);
#5091=ADVANCED_FACE('',(#357),#4855,.T.);
#5092=ADVANCED_FACE('',(#358,#199),#240,.F.);
#5093=ADVANCED_FACE('',(#359,#200),#241,.T.);
#5094=ADVANCED_FACE('',(#360),#4856,.T.);
#5095=ADVANCED_FACE('',(#361),#4857,.T.);
#5096=ADVANCED_FACE('',(#362),#4858,.T.);
#5097=ADVANCED_FACE('',(#363),#4859,.T.);
#5098=ADVANCED_FACE('',(#364),#4860,.F.);
#5099=ADVANCED_FACE('',(#365),#4861,.F.);
#5100=ADVANCED_FACE('',(#366),#4862,.T.);
#5101=ADVANCED_FACE('',(#367),#4863,.T.);
#5102=ADVANCED_FACE('',(#368),#4864,.F.);
#5103=ADVANCED_FACE('',(#369),#4865,.T.);
#5104=ADVANCED_FACE('',(#370),#4866,.F.);
#5105=ADVANCED_FACE('',(#371),#4867,.T.);
#5106=ADVANCED_FACE('',(#372),#4868,.T.);
#5107=ADVANCED_FACE('',(#373),#4869,.F.);
#5108=ADVANCED_FACE('',(#374),#4870,.T.);
#5109=ADVANCED_FACE('',(#375),#4871,.T.);
#5110=ADVANCED_FACE('',(#376),#4872,.T.);
#5111=ADVANCED_FACE('',(#377),#4873,.F.);
#5112=ADVANCED_FACE('',(#378),#4874,.T.);
#5113=ADVANCED_FACE('',(#379),#4875,.T.);
#5114=ADVANCED_FACE('',(#380),#4876,.T.);
#5115=ADVANCED_FACE('',(#381),#4877,.F.);
#5116=ADVANCED_FACE('',(#382),#4878,.T.);
#5117=ADVANCED_FACE('',(#383),#4879,.T.);
#5118=ADVANCED_FACE('',(#384),#4880,.T.);
#5119=ADVANCED_FACE('',(#385),#4881,.F.);
#5120=ADVANCED_FACE('',(#386),#4882,.T.);
#5121=ADVANCED_FACE('',(#387),#4883,.T.);
#5122=ADVANCED_FACE('',(#388),#4884,.T.);
#5123=ADVANCED_FACE('',(#389),#4885,.F.);
#5124=ADVANCED_FACE('',(#390),#4886,.T.);
#5125=ADVANCED_FACE('',(#391),#4887,.T.);
#5126=ADVANCED_FACE('',(#392),#4888,.T.);
#5127=ADVANCED_FACE('',(#393),#4889,.T.);
#5128=ADVANCED_FACE('',(#394),#4890,.F.);
#5129=ADVANCED_FACE('',(#395),#4891,.T.);
#5130=ADVANCED_FACE('',(#396),#4892,.T.);
#5131=ADVANCED_FACE('',(#397),#4893,.T.);
#5132=ADVANCED_FACE('',(#398),#4894,.F.);
#5133=ADVANCED_FACE('',(#399),#4895,.T.);
#5134=ADVANCED_FACE('',(#400),#4896,.T.);
#5135=ADVANCED_FACE('',(#401),#4897,.T.);
#5136=ADVANCED_FACE('',(#402),#4898,.F.);
#5137=ADVANCED_FACE('',(#403),#4899,.T.);
#5138=ADVANCED_FACE('',(#404),#4900,.T.);
#5139=ADVANCED_FACE('',(#405),#4901,.T.);
#5140=ADVANCED_FACE('',(#406),#4902,.F.);
#5141=ADVANCED_FACE('',(#407),#4903,.T.);
#5142=ADVANCED_FACE('',(#408),#4904,.T.);
#5143=ADVANCED_FACE('',(#409),#4905,.T.);
#5144=ADVANCED_FACE('',(#410),#4906,.F.);
#5145=ADVANCED_FACE('',(#411),#4907,.T.);
#5146=ADVANCED_FACE('',(#412),#4908,.T.);
#5147=ADVANCED_FACE('',(#413),#4909,.F.);
#5148=ADVANCED_FACE('',(#414),#4910,.T.);
#5149=ADVANCED_FACE('',(#415),#4911,.T.);
#5150=ADVANCED_FACE('',(#416),#4912,.F.);
#5151=ADVANCED_FACE('',(#417),#4913,.T.);
#5152=ADVANCED_FACE('',(#418),#4914,.F.);
#5153=ADVANCED_FACE('',(#419),#4915,.T.);
#5154=ADVANCED_FACE('',(#420),#4916,.T.);
#5155=ADVANCED_FACE('',(#421),#4917,.F.);
#5156=ADVANCED_FACE('',(#422),#4918,.T.);
#5157=ADVANCED_FACE('',(#423),#4919,.T.);
#5158=ADVANCED_FACE('',(#424),#4920,.T.);
#5159=ADVANCED_FACE('',(#425),#4921,.F.);
#5160=ADVANCED_FACE('',(#426),#4922,.T.);
#5161=ADVANCED_FACE('',(#427),#4923,.F.);
#5162=ADVANCED_FACE('',(#428),#4924,.T.);
#5163=ADVANCED_FACE('',(#429),#4925,.T.);
#5164=ADVANCED_FACE('',(#430),#4926,.F.);
#5165=ADVANCED_FACE('',(#431),#4927,.T.);
#5166=ADVANCED_FACE('',(#432),#4928,.F.);
#5167=ADVANCED_FACE('',(#433),#4929,.T.);
#5168=ADVANCED_FACE('',(#434),#4930,.T.);
#5169=ADVANCED_FACE('',(#435),#4931,.F.);
#5170=ADVANCED_FACE('',(#436),#4932,.T.);
#5171=ADVANCED_FACE('',(#437),#4933,.F.);
#5172=ADVANCED_FACE('',(#438),#4934,.T.);
#5173=ADVANCED_FACE('',(#439),#4935,.T.);
#5174=ADVANCED_FACE('',(#440),#4936,.F.);
#5175=ADVANCED_FACE('',(#441),#4937,.T.);
#5176=ADVANCED_FACE('',(#442),#4938,.F.);
#5177=ADVANCED_FACE('',(#443),#4939,.T.);
#5178=ADVANCED_FACE('',(#444),#4940,.T.);
#5179=ADVANCED_FACE('',(#445),#4941,.F.);
#5180=ADVANCED_FACE('',(#446),#4942,.T.);
#5181=ADVANCED_FACE('',(#447),#4943,.F.);
#5182=ADVANCED_FACE('',(#448),#4944,.T.);
#5183=ADVANCED_FACE('',(#449),#4945,.T.);
#5184=ADVANCED_FACE('',(#450),#4946,.F.);
#5185=ADVANCED_FACE('',(#451),#4947,.T.);
#5186=ADVANCED_FACE('',(#452),#4948,.F.);
#5187=ADVANCED_FACE('',(#453),#4949,.T.);
#5188=ADVANCED_FACE('',(#454),#4950,.T.);
#5189=ADVANCED_FACE('',(#455),#4951,.F.);
#5190=ADVANCED_FACE('',(#456),#4952,.T.);
#5191=ADVANCED_FACE('',(#457),#4953,.F.);
#5192=ADVANCED_FACE('',(#458),#4954,.T.);
#5193=ADVANCED_FACE('',(#459),#4955,.T.);
#5194=ADVANCED_FACE('',(#460),#4956,.F.);
#5195=ADVANCED_FACE('',(#461),#4957,.T.);
#5196=ADVANCED_FACE('',(#462),#4958,.F.);
#5197=ADVANCED_FACE('',(#463),#4959,.T.);
#5198=ADVANCED_FACE('',(#464),#4960,.T.);
#5199=ADVANCED_FACE('',(#465),#4961,.F.);
#5200=ADVANCED_FACE('',(#466),#4962,.T.);
#5201=ADVANCED_FACE('',(#467),#4963,.F.);
#5202=ADVANCED_FACE('',(#468),#4964,.T.);
#5203=ADVANCED_FACE('',(#469),#4965,.T.);
#5204=ADVANCED_FACE('',(#470),#4966,.F.);
#5205=ADVANCED_FACE('',(#471),#4967,.T.);
#5206=ADVANCED_FACE('',(#472),#4968,.F.);
#5207=ADVANCED_FACE('',(#473),#4969,.T.);
#5208=ADVANCED_FACE('',(#474),#4970,.T.);
#5209=ADVANCED_FACE('',(#475),#4971,.F.);
#5210=ADVANCED_FACE('',(#476),#4972,.T.);
#5211=ADVANCED_FACE('',(#477),#4973,.F.);
#5212=ADVANCED_FACE('',(#478),#4974,.T.);
#5213=ADVANCED_FACE('',(#479),#4975,.T.);
#5214=ADVANCED_FACE('',(#480),#4976,.F.);
#5215=ADVANCED_FACE('',(#481),#4977,.T.);
#5216=ADVANCED_FACE('',(#482),#4978,.F.);
#5217=ADVANCED_FACE('',(#483),#4979,.T.);
#5218=ADVANCED_FACE('',(#484),#4980,.T.);
#5219=ADVANCED_FACE('',(#485),#4981,.F.);
#5220=ADVANCED_FACE('',(#486),#4982,.T.);
#5221=ADVANCED_FACE('',(#487),#4983,.F.);
#5222=ADVANCED_FACE('',(#488),#4984,.T.);
#5223=ADVANCED_FACE('',(#489),#4985,.T.);
#5224=ADVANCED_FACE('',(#490),#4986,.F.);
#5225=ADVANCED_FACE('',(#491),#4987,.T.);
#5226=ADVANCED_FACE('',(#492),#4988,.F.);
#5227=ADVANCED_FACE('',(#493),#242,.F.);
#5228=ADVANCED_FACE('',(#494),#243,.F.);
#5229=ADVANCED_FACE('',(#495),#244,.F.);
#5301=CLOSED_SHELL('',(#5044,#5045,#5046,#5047,#5048,#5049,#5050,#5051,
#5052,#5053,#5054,#5055,#5056,#5057,#5058,#5059,#5060,#5061,#5062,#5063,
#5064,#5065,#5066,#5067,#5068,#5069,#5070,#5071,#5072,#5073,#5074,#5075,
#5076,#5077,#5078,#5079,#5080,#5081,#5082,#5083,#5084,#5085,#5086,#5087,
#5088,#5089,#5090,#5091,#5092,#5093,#5094,#5095,#5096,#5097,#5098,#5099,
#5100,#5101,#5102,#5103,#5104,#5105,#5106,#5107,#5108,#5109,#5110,#5111,
#5112,#5113,#5114,#5115,#5116,#5117,#5118,#5119,#5120,#5121,#5122,#5123,
#5124,#5125,#5126,#5127,#5128,#5129,#5130,#5131,#5132,#5133,#5134,#5135,
#5136,#5137,#5138,#5139,#5140,#5141,#5142,#5143,#5144,#5145,#5146,#5147,
#5148,#5149,#5150,#5151,#5152,#5153,#5154,#5155,#5156,#5157,#5158,#5159,
#5160,#5161,#5162,#5163,#5164,#5165,#5166,#5167,#5168,#5169,#5170,#5171,
#5172,#5173,#5174,#5175,#5176,#5177,#5178,#5179,#5180,#5181,#5182,#5183,
#5184,#5185,#5186,#5187,#5188,#5189,#5190,#5191,#5192,#5193,#5194,#5195,
#5196,#5197,#5198,#5199,#5200,#5201,#5202,#5203,#5204,#5205,#5206,#5207,
#5208,#5209,#5210,#5211,#5212,#5213,#5214,#5215,#5216,#5217,#5218,#5219,
#5220,#5221,#5222,#5223,#5224,#5225,#5226,#5227,#5228,#5229));
#5466=AXIS2_PLACEMENT_3D('',#8113,#6334,#6335);
#5467=AXIS2_PLACEMENT_3D('',#8114,#6336,#6337);
#5468=AXIS2_PLACEMENT_3D('',#8117,#6338,#6339);
#5469=AXIS2_PLACEMENT_3D('',#8121,#6341,#6342);
#5470=AXIS2_PLACEMENT_3D('',#8123,#6344,#6345);
#5471=AXIS2_PLACEMENT_3D('',#8126,#6346,#6347);
#5472=AXIS2_PLACEMENT_3D('',#8130,#6349,#6350);
#5473=AXIS2_PLACEMENT_3D('',#8132,#6352,#6353);
#5474=AXIS2_PLACEMENT_3D('',#8134,#6354,#6355);
#5475=AXIS2_PLACEMENT_3D('',#8137,#6357,#6358);
#5476=AXIS2_PLACEMENT_3D('',#8138,#6359,#6360);
#5477=AXIS2_PLACEMENT_3D('',#8141,#6361,#6362);
#5478=AXIS2_PLACEMENT_3D('',#8145,#6364,#6365);
#5479=AXIS2_PLACEMENT_3D('',#8147,#6367,#6368);
#5480=AXIS2_PLACEMENT_3D('',#8149,#6369,#6370);
#5481=AXIS2_PLACEMENT_3D('',#8152,#6372,#6373);
#5482=AXIS2_PLACEMENT_3D('',#8153,#6374,#6375);
#5483=AXIS2_PLACEMENT_3D('',#8156,#6376,#6377);
#5484=AXIS2_PLACEMENT_3D('',#8160,#6379,#6380);
#5485=AXIS2_PLACEMENT_3D('',#8162,#6382,#6383);
#5486=AXIS2_PLACEMENT_3D('',#8164,#6384,#6385);
#5487=AXIS2_PLACEMENT_3D('',#8166,#6386,#6387);
#5488=AXIS2_PLACEMENT_3D('',#8168,#6389,#6390);
#5489=AXIS2_PLACEMENT_3D('',#8171,#6391,#6392);
#5490=AXIS2_PLACEMENT_3D('',#8175,#6394,#6395);
#5491=AXIS2_PLACEMENT_3D('',#8177,#6397,#6398);
#5492=AXIS2_PLACEMENT_3D('',#8179,#6399,#6400);
#5493=AXIS2_PLACEMENT_3D('',#8181,#6401,#6402);
#5494=AXIS2_PLACEMENT_3D('',#8183,#6404,#6405);
#5495=AXIS2_PLACEMENT_3D('',#8186,#6406,#6407);
#5496=AXIS2_PLACEMENT_3D('',#8190,#6409,#6410);
#5497=AXIS2_PLACEMENT_3D('',#8192,#6412,#6413);
#5498=AXIS2_PLACEMENT_3D('',#8195,#6414,#6415);
#5499=AXIS2_PLACEMENT_3D('',#8199,#6417,#6418);
#5500=AXIS2_PLACEMENT_3D('',#8201,#6420,#6421);
#5501=AXIS2_PLACEMENT_3D('',#8204,#6422,#6423);
#5502=AXIS2_PLACEMENT_3D('',#8208,#6425,#6426);
#5503=AXIS2_PLACEMENT_3D('',#8210,#6428,#6429);
#5504=AXIS2_PLACEMENT_3D('',#8213,#6430,#6431);
#5505=AXIS2_PLACEMENT_3D('',#8217,#6433,#6434);
#5506=AXIS2_PLACEMENT_3D('',#8219,#6436,#6437);
#5507=AXIS2_PLACEMENT_3D('',#8222,#6438,#6439);
#5508=AXIS2_PLACEMENT_3D('',#8226,#6441,#6442);
#5509=AXIS2_PLACEMENT_3D('',#8228,#6444,#6445);
#5510=AXIS2_PLACEMENT_3D('',#8231,#6446,#6447);
#5511=AXIS2_PLACEMENT_3D('',#8235,#6449,#6450);
#5512=AXIS2_PLACEMENT_3D('',#8237,#6452,#6453);
#5513=AXIS2_PLACEMENT_3D('',#8240,#6454,#6455);
#5514=AXIS2_PLACEMENT_3D('',#8244,#6457,#6458);
#5515=AXIS2_PLACEMENT_3D('',#8246,#6460,#6461);
#5516=AXIS2_PLACEMENT_3D('',#8249,#6462,#6463);
#5517=AXIS2_PLACEMENT_3D('',#8253,#6465,#6466);
#5518=AXIS2_PLACEMENT_3D('',#8255,#6468,#6469);
#5519=AXIS2_PLACEMENT_3D('',#8258,#6470,#6471);
#5520=AXIS2_PLACEMENT_3D('',#8262,#6473,#6474);
#5521=AXIS2_PLACEMENT_3D('',#8264,#6476,#6477);
#5522=AXIS2_PLACEMENT_3D('',#8267,#6478,#6479);
#5523=AXIS2_PLACEMENT_3D('',#8271,#6481,#6482);
#5524=AXIS2_PLACEMENT_3D('',#8273,#6484,#6485);
#5525=AXIS2_PLACEMENT_3D('',#8276,#6486,#6487);
#5526=AXIS2_PLACEMENT_3D('',#8280,#6489,#6490);
#5527=AXIS2_PLACEMENT_3D('',#8282,#6492,#6493);
#5528=AXIS2_PLACEMENT_3D('',#8285,#6494,#6495);
#5529=AXIS2_PLACEMENT_3D('',#8289,#6497,#6498);
#5530=AXIS2_PLACEMENT_3D('',#8291,#6500,#6501);
#5531=AXIS2_PLACEMENT_3D('',#8294,#6502,#6503);
#5532=AXIS2_PLACEMENT_3D('',#8298,#6505,#6506);
#5533=AXIS2_PLACEMENT_3D('',#8300,#6508,#6509);
#5534=AXIS2_PLACEMENT_3D('',#8303,#6510,#6511);
#5535=AXIS2_PLACEMENT_3D('',#8307,#6513,#6514);
#5536=AXIS2_PLACEMENT_3D('',#8309,#6516,#6517);
#5537=AXIS2_PLACEMENT_3D('',#8312,#6518,#6519);
#5538=AXIS2_PLACEMENT_3D('',#8316,#6521,#6522);
#5539=AXIS2_PLACEMENT_3D('',#8318,#6524,#6525);
#5540=AXIS2_PLACEMENT_3D('',#8321,#6526,#6527);
#5541=AXIS2_PLACEMENT_3D('',#8325,#6529,#6530);
#5542=AXIS2_PLACEMENT_3D('',#8327,#6532,#6533);
#5543=AXIS2_PLACEMENT_3D('',#8330,#6534,#6535);
#5544=AXIS2_PLACEMENT_3D('',#8334,#6537,#6538);
#5545=AXIS2_PLACEMENT_3D('',#8336,#6540,#6541);
#5546=AXIS2_PLACEMENT_3D('',#8339,#6542,#6543);
#5547=AXIS2_PLACEMENT_3D('',#8343,#6545,#6546);
#5548=AXIS2_PLACEMENT_3D('',#8345,#6548,#6549);
#5549=AXIS2_PLACEMENT_3D('',#8348,#6550,#6551);
#5550=AXIS2_PLACEMENT_3D('',#8352,#6553,#6554);
#5551=AXIS2_PLACEMENT_3D('',#8354,#6556,#6557);
#5552=AXIS2_PLACEMENT_3D('',#8357,#6558,#6559);
#5553=AXIS2_PLACEMENT_3D('',#8361,#6561,#6562);
#5554=AXIS2_PLACEMENT_3D('',#8363,#6564,#6565);
#5555=AXIS2_PLACEMENT_3D('',#8366,#6566,#6567);
#5556=AXIS2_PLACEMENT_3D('',#8370,#6569,#6570);
#5557=AXIS2_PLACEMENT_3D('',#8372,#6572,#6573);
#5558=AXIS2_PLACEMENT_3D('',#8375,#6574,#6575);
#5559=AXIS2_PLACEMENT_3D('',#8379,#6577,#6578);
#5560=AXIS2_PLACEMENT_3D('',#8381,#6580,#6581);
#5561=AXIS2_PLACEMENT_3D('',#8384,#6582,#6583);
#5562=AXIS2_PLACEMENT_3D('',#8388,#6585,#6586);
#5563=AXIS2_PLACEMENT_3D('',#8390,#6588,#6589);
#5564=AXIS2_PLACEMENT_3D('',#8393,#6590,#6591);
#5565=AXIS2_PLACEMENT_3D('',#8397,#6593,#6594);
#5566=AXIS2_PLACEMENT_3D('',#8399,#6596,#6597);
#5567=AXIS2_PLACEMENT_3D('',#8401,#6598,#6599);
#5568=AXIS2_PLACEMENT_3D('',#8404,#6601,#6602);
#5569=AXIS2_PLACEMENT_3D('',#8405,#6603,#6604);
#5570=AXIS2_PLACEMENT_3D('',#8407,#6605,#6606);
#5571=AXIS2_PLACEMENT_3D('',#8410,#6608,#6609);
#5572=AXIS2_PLACEMENT_3D('',#8411,#6610,#6611);
#5573=AXIS2_PLACEMENT_3D('',#8413,#6612,#6613);
#5574=AXIS2_PLACEMENT_3D('',#8416,#6615,#6616);
#5575=AXIS2_PLACEMENT_3D('',#8417,#6617,#6618);
#5576=AXIS2_PLACEMENT_3D('',#8420,#6619,#6620);
#5577=AXIS2_PLACEMENT_3D('',#8424,#6622,#6623);
#5578=AXIS2_PLACEMENT_3D('',#8426,#6625,#6626);
#5579=AXIS2_PLACEMENT_3D('',#8429,#6627,#6628);
#5580=AXIS2_PLACEMENT_3D('',#8433,#6630,#6631);
#5581=AXIS2_PLACEMENT_3D('',#8435,#6633,#6634);
#5582=AXIS2_PLACEMENT_3D('',#8438,#6635,#6636);
#5583=AXIS2_PLACEMENT_3D('',#8442,#6638,#6639);
#5584=AXIS2_PLACEMENT_3D('',#8444,#6641,#6642);
#5585=AXIS2_PLACEMENT_3D('',#8447,#6643,#6644);
#5586=AXIS2_PLACEMENT_3D('',#8451,#6646,#6647);
#5587=AXIS2_PLACEMENT_3D('',#8453,#6649,#6650);
#5588=AXIS2_PLACEMENT_3D('',#8456,#6651,#6652);
#5589=AXIS2_PLACEMENT_3D('',#8460,#6654,#6655);
#5590=AXIS2_PLACEMENT_3D('',#8462,#6657,#6658);
#5591=AXIS2_PLACEMENT_3D('',#8465,#6659,#6660);
#5592=AXIS2_PLACEMENT_3D('',#8469,#6662,#6663);
#5593=AXIS2_PLACEMENT_3D('',#8471,#6665,#6666);
#5594=AXIS2_PLACEMENT_3D('',#8474,#6667,#6668);
#5595=AXIS2_PLACEMENT_3D('',#8478,#6670,#6671);
#5596=AXIS2_PLACEMENT_3D('',#8480,#6673,#6674);
#5597=AXIS2_PLACEMENT_3D('',#8483,#6675,#6676);
#5598=AXIS2_PLACEMENT_3D('',#8487,#6678,#6679);
#5599=AXIS2_PLACEMENT_3D('',#8489,#6681,#6682);
#5600=AXIS2_PLACEMENT_3D('',#8492,#6683,#6684);
#5601=AXIS2_PLACEMENT_3D('',#8496,#6686,#6687);
#5602=AXIS2_PLACEMENT_3D('',#8498,#6689,#6690);
#5603=AXIS2_PLACEMENT_3D('',#8501,#6691,#6692);
#5604=AXIS2_PLACEMENT_3D('',#8505,#6694,#6695);
#5605=AXIS2_PLACEMENT_3D('',#8507,#6697,#6698);
#5606=AXIS2_PLACEMENT_3D('',#8510,#6699,#6700);
#5607=AXIS2_PLACEMENT_3D('',#8514,#6702,#6703);
#5608=AXIS2_PLACEMENT_3D('',#8516,#6705,#6706);
#5609=AXIS2_PLACEMENT_3D('',#8519,#6707,#6708);
#5610=AXIS2_PLACEMENT_3D('',#8523,#6710,#6711);
#5611=AXIS2_PLACEMENT_3D('',#8525,#6713,#6714);
#5612=AXIS2_PLACEMENT_3D('',#8527,#6715,#6716);
#5613=AXIS2_PLACEMENT_3D('',#8529,#6717,#6718);
#5614=AXIS2_PLACEMENT_3D('',#8531,#6719,#6720);
#5615=AXIS2_PLACEMENT_3D('',#8533,#6721,#6722);
#5616=AXIS2_PLACEMENT_3D('',#8534,#6723,#6724);
#5617=AXIS2_PLACEMENT_3D('',#8536,#6725,#6726);
#5618=AXIS2_PLACEMENT_3D('',#8538,#6727,#6728);
#5619=AXIS2_PLACEMENT_3D('',#8540,#6729,#6730);
#5620=AXIS2_PLACEMENT_3D('',#8542,#6731,#6732);
#5621=AXIS2_PLACEMENT_3D('',#8543,#6733,#6734);
#5622=AXIS2_PLACEMENT_3D('',#8545,#6735,#6736);
#5623=AXIS2_PLACEMENT_3D('',#8547,#6737,#6738);
#5624=AXIS2_PLACEMENT_3D('',#8549,#6739,#6740);
#5625=AXIS2_PLACEMENT_3D('',#8551,#6741,#6742);
#5626=AXIS2_PLACEMENT_3D('',#8552,#6743,#6744);
#5627=AXIS2_PLACEMENT_3D('',#8554,#6745,#6746);
#5628=AXIS2_PLACEMENT_3D('',#8556,#6747,#6748);
#5629=AXIS2_PLACEMENT_3D('',#8558,#6749,#6750);
#5630=AXIS2_PLACEMENT_3D('',#8560,#6751,#6752);
#5631=AXIS2_PLACEMENT_3D('',#8561,#6753,#6754);
#5632=AXIS2_PLACEMENT_3D('',#8563,#6755,#6756);
#5633=AXIS2_PLACEMENT_3D('',#8565,#6757,#6758);
#5634=AXIS2_PLACEMENT_3D('',#8567,#6759,#6760);
#5635=AXIS2_PLACEMENT_3D('',#8569,#6761,#6762);
#5636=AXIS2_PLACEMENT_3D('',#8570,#6763,#6764);
#5637=AXIS2_PLACEMENT_3D('',#8572,#6765,#6766);
#5638=AXIS2_PLACEMENT_3D('',#8574,#6767,#6768);
#5639=AXIS2_PLACEMENT_3D('',#8576,#6769,#6770);
#5640=AXIS2_PLACEMENT_3D('',#8578,#6771,#6772);
#5641=AXIS2_PLACEMENT_3D('',#8579,#6773,#6774);
#5642=AXIS2_PLACEMENT_3D('',#8581,#6775,#6776);
#5643=AXIS2_PLACEMENT_3D('',#8583,#6777,#6778);
#5644=AXIS2_PLACEMENT_3D('',#8585,#6779,#6780);
#5645=AXIS2_PLACEMENT_3D('',#8587,#6781,#6782);
#5646=AXIS2_PLACEMENT_3D('',#8588,#6783,#6784);
#5647=AXIS2_PLACEMENT_3D('',#8590,#6785,#6786);
#5648=AXIS2_PLACEMENT_3D('',#8592,#6787,#6788);
#5649=AXIS2_PLACEMENT_3D('',#8594,#6789,#6790);
#5650=AXIS2_PLACEMENT_3D('',#8596,#6791,#6792);
#5651=AXIS2_PLACEMENT_3D('',#8597,#6793,#6794);
#5652=AXIS2_PLACEMENT_3D('',#8599,#6795,#6796);
#5653=AXIS2_PLACEMENT_3D('',#8601,#6797,#6798);
#5654=AXIS2_PLACEMENT_3D('',#8603,#6799,#6800);
#5655=AXIS2_PLACEMENT_3D('',#8605,#6801,#6802);
#5656=AXIS2_PLACEMENT_3D('',#8606,#6803,#6804);
#5657=AXIS2_PLACEMENT_3D('',#8608,#6805,#6806);
#5658=AXIS2_PLACEMENT_3D('',#8610,#6807,#6808);
#5659=AXIS2_PLACEMENT_3D('',#8612,#6809,#6810);
#5660=AXIS2_PLACEMENT_3D('',#8614,#6811,#6812);
#5661=AXIS2_PLACEMENT_3D('',#8615,#6813,#6814);
#5662=AXIS2_PLACEMENT_3D('',#8617,#6815,#6816);
#5663=AXIS2_PLACEMENT_3D('',#8619,#6817,#6818);
#5664=AXIS2_PLACEMENT_3D('',#8621,#6819,#6820);
#5665=AXIS2_PLACEMENT_3D('',#8623,#6821,#6822);
#5666=AXIS2_PLACEMENT_3D('',#8624,#6823,#6824);
#5667=AXIS2_PLACEMENT_3D('',#8626,#6825,#6826);
#5668=AXIS2_PLACEMENT_3D('',#8628,#6827,#6828);
#5669=AXIS2_PLACEMENT_3D('',#8630,#6829,#6830);
#5670=AXIS2_PLACEMENT_3D('',#8632,#6831,#6832);
#5671=AXIS2_PLACEMENT_3D('',#8633,#6833,#6834);
#5672=AXIS2_PLACEMENT_3D('',#8635,#6835,#6836);
#5673=AXIS2_PLACEMENT_3D('',#8637,#6837,#6838);
#5674=AXIS2_PLACEMENT_3D('',#8638,#6839,#6840);
#5675=AXIS2_PLACEMENT_3D('',#8640,#6841,#6842);
#5676=AXIS2_PLACEMENT_3D('',#8642,#6843,#6844);
#5677=AXIS2_PLACEMENT_3D('',#8643,#6845,#6846);
#5678=AXIS2_PLACEMENT_3D('',#8644,#6847,#6848);
#5679=AXIS2_PLACEMENT_3D('',#8646,#6849,#6850);
#5680=AXIS2_PLACEMENT_3D('',#8648,#6851,#6852);
#5681=AXIS2_PLACEMENT_3D('',#8649,#6853,#6854);
#5682=AXIS2_PLACEMENT_3D('',#8650,#6855,#6856);
#5683=AXIS2_PLACEMENT_3D('',#8652,#6857,#6858);
#5684=AXIS2_PLACEMENT_3D('',#8654,#6859,#6860);
#5685=AXIS2_PLACEMENT_3D('',#8655,#6861,#6862);
#5686=AXIS2_PLACEMENT_3D('',#8656,#6863,#6864);
#5687=AXIS2_PLACEMENT_3D('',#8658,#6865,#6866);
#5688=AXIS2_PLACEMENT_3D('',#8660,#6867,#6868);
#5689=AXIS2_PLACEMENT_3D('',#8661,#6869,#6870);
#5690=AXIS2_PLACEMENT_3D('',#8662,#6871,#6872);
#5691=AXIS2_PLACEMENT_3D('',#8664,#6873,#6874);
#5692=AXIS2_PLACEMENT_3D('',#8666,#6875,#6876);
#5693=AXIS2_PLACEMENT_3D('',#8667,#6877,#6878);
#5694=AXIS2_PLACEMENT_3D('',#8668,#6879,#6880);
#5695=AXIS2_PLACEMENT_3D('',#8670,#6881,#6882);
#5696=AXIS2_PLACEMENT_3D('',#8672,#6883,#6884);
#5697=AXIS2_PLACEMENT_3D('',#8673,#6885,#6886);
#5698=AXIS2_PLACEMENT_3D('',#8675,#6887,#6888);
#5699=AXIS2_PLACEMENT_3D('',#8677,#6889,#6890);
#5700=AXIS2_PLACEMENT_3D('',#8678,#6891,#6892);
#5701=AXIS2_PLACEMENT_3D('',#8679,#6893,#6894);
#5702=AXIS2_PLACEMENT_3D('',#8681,#6895,#6896);
#5703=AXIS2_PLACEMENT_3D('',#8683,#6897,#6898);
#5704=AXIS2_PLACEMENT_3D('',#8684,#6899,#6900);
#5705=AXIS2_PLACEMENT_3D('',#8685,#6901,#6902);
#5706=AXIS2_PLACEMENT_3D('',#8687,#6903,#6904);
#5707=AXIS2_PLACEMENT_3D('',#8689,#6905,#6906);
#5708=AXIS2_PLACEMENT_3D('',#8690,#6907,#6908);
#5709=AXIS2_PLACEMENT_3D('',#8691,#6909,#6910);
#5710=AXIS2_PLACEMENT_3D('',#8693,#6911,#6912);
#5711=AXIS2_PLACEMENT_3D('',#8695,#6913,#6914);
#5712=AXIS2_PLACEMENT_3D('',#8696,#6915,#6916);
#5713=AXIS2_PLACEMENT_3D('',#8697,#6917,#6918);
#5714=AXIS2_PLACEMENT_3D('',#8699,#6919,#6920);
#5715=AXIS2_PLACEMENT_3D('',#8701,#6921,#6922);
#5716=AXIS2_PLACEMENT_3D('',#8702,#6923,#6924);
#5717=AXIS2_PLACEMENT_3D('',#8703,#6925,#6926);
#5718=AXIS2_PLACEMENT_3D('',#8705,#6927,#6928);
#5719=AXIS2_PLACEMENT_3D('',#8707,#6929,#6930);
#5720=AXIS2_PLACEMENT_3D('',#8708,#6931,#6932);
#5721=AXIS2_PLACEMENT_3D('',#8710,#6933,#6934);
#5722=AXIS2_PLACEMENT_3D('',#8712,#6935,#6936);
#5723=AXIS2_PLACEMENT_3D('',#8713,#6937,#6938);
#5724=AXIS2_PLACEMENT_3D('',#8715,#6939,#6940);
#5725=AXIS2_PLACEMENT_3D('',#8717,#6941,#6942);
#5726=AXIS2_PLACEMENT_3D('',#8719,#6943,#6944);
#5727=AXIS2_PLACEMENT_3D('',#8721,#6945,#6946);
#5728=AXIS2_PLACEMENT_3D('',#8723,#6947,#6948);
#5729=AXIS2_PLACEMENT_3D('',#8724,#6949,#6950);
#5730=AXIS2_PLACEMENT_3D('',#8726,#6951,#6952);
#5731=AXIS2_PLACEMENT_3D('',#8728,#6953,#6954);
#5732=AXIS2_PLACEMENT_3D('',#8730,#6955,#6956);
#5733=AXIS2_PLACEMENT_3D('',#8732,#6957,#6958);
#5734=AXIS2_PLACEMENT_3D('',#8733,#6959,#6960);
#5735=AXIS2_PLACEMENT_3D('',#8735,#6961,#6962);
#5736=AXIS2_PLACEMENT_3D('',#8737,#6963,#6964);
#5737=AXIS2_PLACEMENT_3D('',#8739,#6965,#6966);
#5738=AXIS2_PLACEMENT_3D('',#8741,#6967,#6968);
#5739=AXIS2_PLACEMENT_3D('',#8742,#6969,#6970);
#5740=AXIS2_PLACEMENT_3D('',#8744,#6971,#6972);
#5741=AXIS2_PLACEMENT_3D('',#8746,#6973,#6974);
#5742=AXIS2_PLACEMENT_3D('',#8748,#6975,#6976);
#5743=AXIS2_PLACEMENT_3D('',#8750,#6977,#6978);
#5744=AXIS2_PLACEMENT_3D('',#8751,#6979,#6980);
#5745=AXIS2_PLACEMENT_3D('',#8757,#6984,#6985);
#5746=AXIS2_PLACEMENT_3D('',#8759,#6986,#6987);
#5747=AXIS2_PLACEMENT_3D('',#8761,#6988,#6989);
#5748=AXIS2_PLACEMENT_3D('',#8763,#6990,#6991);
#5749=AXIS2_PLACEMENT_3D('',#8765,#6992,#6993);
#5750=AXIS2_PLACEMENT_3D('',#8767,#6994,#6995);
#5751=AXIS2_PLACEMENT_3D('',#8768,#6996,#6997);
#5752=AXIS2_PLACEMENT_3D('',#8770,#6998,#6999);
#5753=AXIS2_PLACEMENT_3D('',#8772,#7000,#7001);
#5754=AXIS2_PLACEMENT_3D('',#8774,#7002,#7003);
#5755=AXIS2_PLACEMENT_3D('',#8776,#7004,#7005);
#5756=AXIS2_PLACEMENT_3D('',#8777,#7006,#7007);
#5757=AXIS2_PLACEMENT_3D('',#8779,#7008,#7009);
#5758=AXIS2_PLACEMENT_3D('',#8781,#7010,#7011);
#5759=AXIS2_PLACEMENT_3D('',#8783,#7012,#7013);
#5760=AXIS2_PLACEMENT_3D('',#8785,#7014,#7015);
#5761=AXIS2_PLACEMENT_3D('',#8786,#7016,#7017);
#5762=AXIS2_PLACEMENT_3D('',#8788,#7018,#7019);
#5763=AXIS2_PLACEMENT_3D('',#8790,#7020,#7021);
#5764=AXIS2_PLACEMENT_3D('',#8792,#7022,#7023);
#5765=AXIS2_PLACEMENT_3D('',#8794,#7024,#7025);
#5766=AXIS2_PLACEMENT_3D('',#8796,#7026,#7027);
#5767=AXIS2_PLACEMENT_3D('',#8797,#7028,#7029);
#5768=AXIS2_PLACEMENT_3D('',#8799,#7030,#7031);
#5769=AXIS2_PLACEMENT_3D('',#8801,#7032,#7033);
#5770=AXIS2_PLACEMENT_3D('',#8802,#7034,#7035);
#5771=AXIS2_PLACEMENT_3D('',#8804,#7036,#7037);
#5772=AXIS2_PLACEMENT_3D('',#8806,#7038,#7039);
#5773=AXIS2_PLACEMENT_3D('',#8807,#7040,#7041);
#5774=AXIS2_PLACEMENT_3D('',#8808,#7042,#7043);
#5775=AXIS2_PLACEMENT_3D('',#8810,#7044,#7045);
#5776=AXIS2_PLACEMENT_3D('',#8812,#7046,#7047);
#5777=AXIS2_PLACEMENT_3D('',#8813,#7048,#7049);
#5778=AXIS2_PLACEMENT_3D('',#8814,#7050,#7051);
#5779=AXIS2_PLACEMENT_3D('',#8816,#7052,#7053);
#5780=AXIS2_PLACEMENT_3D('',#8818,#7054,#7055);
#5781=AXIS2_PLACEMENT_3D('',#8819,#7056,#7057);
#5782=AXIS2_PLACEMENT_3D('',#8820,#7058,#7059);
#5783=AXIS2_PLACEMENT_3D('',#8822,#7060,#7061);
#5784=AXIS2_PLACEMENT_3D('',#8824,#7062,#7063);
#5785=AXIS2_PLACEMENT_3D('',#8825,#7064,#7065);
#5786=AXIS2_PLACEMENT_3D('',#8826,#7066,#7067);
#5787=AXIS2_PLACEMENT_3D('',#8828,#7068,#7069);
#5788=AXIS2_PLACEMENT_3D('',#8830,#7070,#7071);
#5789=AXIS2_PLACEMENT_3D('',#8831,#7072,#7073);
#5790=AXIS2_PLACEMENT_3D('',#8832,#7074,#7075);
#5791=AXIS2_PLACEMENT_3D('',#8834,#7076,#7077);
#5792=AXIS2_PLACEMENT_3D('',#8836,#7078,#7079);
#5793=AXIS2_PLACEMENT_3D('',#8837,#7080,#7081);
#5794=AXIS2_PLACEMENT_3D('',#8839,#7082,#7083);
#5795=AXIS2_PLACEMENT_3D('',#8841,#7084,#7085);
#5796=AXIS2_PLACEMENT_3D('',#8842,#7086,#7087);
#5797=AXIS2_PLACEMENT_3D('',#8843,#7088,#7089);
#5798=AXIS2_PLACEMENT_3D('',#8845,#7090,#7091);
#5799=AXIS2_PLACEMENT_3D('',#8847,#7092,#7093);
#5800=AXIS2_PLACEMENT_3D('',#8848,#7094,#7095);
#5801=AXIS2_PLACEMENT_3D('',#8849,#7096,#7097);
#5802=AXIS2_PLACEMENT_3D('',#8851,#7098,#7099);
#5803=AXIS2_PLACEMENT_3D('',#8853,#7100,#7101);
#5804=AXIS2_PLACEMENT_3D('',#8854,#7102,#7103);
#5805=AXIS2_PLACEMENT_3D('',#8855,#7104,#7105);
#5806=AXIS2_PLACEMENT_3D('',#8857,#7106,#7107);
#5807=AXIS2_PLACEMENT_3D('',#8859,#7108,#7109);
#5808=AXIS2_PLACEMENT_3D('',#8860,#7110,#7111);
#5809=AXIS2_PLACEMENT_3D('',#8861,#7112,#7113);
#5810=AXIS2_PLACEMENT_3D('',#8863,#7114,#7115);
#5811=AXIS2_PLACEMENT_3D('',#8865,#7116,#7117);
#5812=AXIS2_PLACEMENT_3D('',#8866,#7118,#7119);
#5813=AXIS2_PLACEMENT_3D('',#8867,#7120,#7121);
#5814=AXIS2_PLACEMENT_3D('',#8869,#7122,#7123);
#5815=AXIS2_PLACEMENT_3D('',#8871,#7124,#7125);
#5816=AXIS2_PLACEMENT_3D('',#8872,#7126,#7127);
#5817=AXIS2_PLACEMENT_3D('',#8874,#7128,#7129);
#5818=AXIS2_PLACEMENT_3D('',#8876,#7130,#7131);
#5819=AXIS2_PLACEMENT_3D('',#8877,#7132,#7133);
#5820=AXIS2_PLACEMENT_3D('',#8879,#7134,#7135);
#5821=AXIS2_PLACEMENT_3D('',#8881,#7136,#7137);
#5822=AXIS2_PLACEMENT_3D('',#8883,#7138,#7139);
#5823=AXIS2_PLACEMENT_3D('',#8885,#7140,#7141);
#5824=AXIS2_PLACEMENT_3D('',#8886,#7142,#7143);
#5825=AXIS2_PLACEMENT_3D('',#8888,#7144,#7145);
#5826=AXIS2_PLACEMENT_3D('',#8890,#7146,#7147);
#5827=AXIS2_PLACEMENT_3D('',#8892,#7148,#7149);
#5828=AXIS2_PLACEMENT_3D('',#8894,#7150,#7151);
#5829=AXIS2_PLACEMENT_3D('',#8895,#7152,#7153);
#5830=AXIS2_PLACEMENT_3D('',#8897,#7154,#7155);
#5831=AXIS2_PLACEMENT_3D('',#8899,#7156,#7157);
#5832=AXIS2_PLACEMENT_3D('',#8901,#7158,#7159);
#5833=AXIS2_PLACEMENT_3D('',#8903,#7160,#7161);
#5834=AXIS2_PLACEMENT_3D('',#8904,#7162,#7163);
#5835=AXIS2_PLACEMENT_3D('',#8906,#7164,#7165);
#5836=AXIS2_PLACEMENT_3D('',#8908,#7166,#7167);
#5837=AXIS2_PLACEMENT_3D('',#8910,#7168,#7169);
#5838=AXIS2_PLACEMENT_3D('',#8912,#7170,#7171);
#5839=AXIS2_PLACEMENT_3D('',#8913,#7172,#7173);
#5840=AXIS2_PLACEMENT_3D('',#8915,#7174,#7175);
#5841=AXIS2_PLACEMENT_3D('',#8917,#7176,#7177);
#5842=AXIS2_PLACEMENT_3D('',#8919,#7178,#7179);
#5843=AXIS2_PLACEMENT_3D('',#8921,#7180,#7181);
#5844=AXIS2_PLACEMENT_3D('',#8922,#7182,#7183);
#5845=AXIS2_PLACEMENT_3D('',#8924,#7184,#7185);
#5846=AXIS2_PLACEMENT_3D('',#8926,#7186,#7187);
#5847=AXIS2_PLACEMENT_3D('',#8928,#7188,#7189);
#5848=AXIS2_PLACEMENT_3D('',#8930,#7190,#7191);
#5849=AXIS2_PLACEMENT_3D('',#8931,#7192,#7193);
#5850=AXIS2_PLACEMENT_3D('',#8933,#7194,#7195);
#5851=AXIS2_PLACEMENT_3D('',#8935,#7196,#7197);
#5852=AXIS2_PLACEMENT_3D('',#8937,#7198,#7199);
#5853=AXIS2_PLACEMENT_3D('',#8939,#7200,#7201);
#5854=AXIS2_PLACEMENT_3D('',#8940,#7202,#7203);
#5855=AXIS2_PLACEMENT_3D('',#8942,#7204,#7205);
#5856=AXIS2_PLACEMENT_3D('',#8944,#7206,#7207);
#5857=AXIS2_PLACEMENT_3D('',#8946,#7208,#7209);
#5858=AXIS2_PLACEMENT_3D('',#8948,#7210,#7211);
#5859=AXIS2_PLACEMENT_3D('',#8949,#7212,#7213);
#5860=AXIS2_PLACEMENT_3D('',#8951,#7214,#7215);
#5861=AXIS2_PLACEMENT_3D('',#8953,#7216,#7217);
#5862=AXIS2_PLACEMENT_3D('',#8955,#7218,#7219);
#5863=AXIS2_PLACEMENT_3D('',#8957,#7220,#7221);
#5864=AXIS2_PLACEMENT_3D('',#8958,#7222,#7223);
#5865=AXIS2_PLACEMENT_3D('',#8960,#7224,#7225);
#5866=AXIS2_PLACEMENT_3D('',#8962,#7226,#7227);
#5867=AXIS2_PLACEMENT_3D('',#8964,#7228,#7229);
#5868=AXIS2_PLACEMENT_3D('',#8966,#7230,#7231);
#5869=AXIS2_PLACEMENT_3D('',#8967,#7232,#7233);
#5870=AXIS2_PLACEMENT_3D('',#8969,#7234,#7235);
#5871=AXIS2_PLACEMENT_3D('',#8971,#7236,#7237);
#5872=AXIS2_PLACEMENT_3D('',#8973,#7238,#7239);
#5873=AXIS2_PLACEMENT_3D('',#8975,#7240,#7241);
#5874=AXIS2_PLACEMENT_3D('',#8976,#7242,#7243);
#5875=AXIS2_PLACEMENT_3D('',#8978,#7244,#7245);
#5876=AXIS2_PLACEMENT_3D('',#8980,#7246,#7247);
#5877=AXIS2_PLACEMENT_3D('',#8982,#7248,#7249);
#5878=AXIS2_PLACEMENT_3D('',#8983,#7250,#7251);
#5879=AXIS2_PLACEMENT_3D('',#8989,#7255,#7256);
#5880=AXIS2_PLACEMENT_3D('',#8991,#7258,#7259);
#5881=AXIS2_PLACEMENT_3D('',#8993,#7261,#7262);
#5882=AXIS2_PLACEMENT_3D('',#8995,#7264,#7265);
#5883=AXIS2_PLACEMENT_3D('',#8998,#7268,#7269);
#5884=AXIS2_PLACEMENT_3D('',#8999,#7270,#7271);
#5885=AXIS2_PLACEMENT_3D('',#9000,#7272,#7273);
#5886=AXIS2_PLACEMENT_3D('',#9002,#7275,#7276);
#5887=AXIS2_PLACEMENT_3D('',#9004,#7278,#7279);
#5888=AXIS2_PLACEMENT_3D('',#9006,#7281,#7282);
#5889=AXIS2_PLACEMENT_3D('',#9008,#7284,#7285);
#5890=AXIS2_PLACEMENT_3D('',#9009,#7286,#7287);
#5891=AXIS2_PLACEMENT_3D('',#9010,#7288,#7289);
#5892=AXIS2_PLACEMENT_3D('',#9012,#7291,#7292);
#5893=AXIS2_PLACEMENT_3D('',#9014,#7294,#7295);
#5894=AXIS2_PLACEMENT_3D('',#9015,#7296,#7297);
#5895=AXIS2_PLACEMENT_3D('',#9016,#7298,#7299);
#5896=AXIS2_PLACEMENT_3D('',#9018,#7301,#7302);
#5897=AXIS2_PLACEMENT_3D('',#9020,#7304,#7305);
#5898=AXIS2_PLACEMENT_3D('',#9021,#7306,#7307);
#5899=AXIS2_PLACEMENT_3D('',#9022,#7308,#7309);
#5900=AXIS2_PLACEMENT_3D('',#9024,#7311,#7312);
#5901=AXIS2_PLACEMENT_3D('',#9026,#7314,#7315);
#5902=AXIS2_PLACEMENT_3D('',#9027,#7316,#7317);
#5903=AXIS2_PLACEMENT_3D('',#9028,#7318,#7319);
#5904=AXIS2_PLACEMENT_3D('',#9030,#7321,#7322);
#5905=AXIS2_PLACEMENT_3D('',#9032,#7324,#7325);
#5906=AXIS2_PLACEMENT_3D('',#9033,#7326,#7327);
#5907=AXIS2_PLACEMENT_3D('',#9034,#7328,#7329);
#5908=AXIS2_PLACEMENT_3D('',#9036,#7331,#7332);
#5909=AXIS2_PLACEMENT_3D('',#9038,#7334,#7335);
#5910=AXIS2_PLACEMENT_3D('',#9039,#7336,#7337);
#5911=AXIS2_PLACEMENT_3D('',#9041,#7339,#7340);
#5912=AXIS2_PLACEMENT_3D('',#9042,#7341,#7342);
#5913=AXIS2_PLACEMENT_3D('',#9044,#7344,#7345);
#5914=AXIS2_PLACEMENT_3D('',#9045,#7346,#7347);
#5915=AXIS2_PLACEMENT_3D('',#9047,#7349,#7350);
#5916=AXIS2_PLACEMENT_3D('',#9048,#7351,#7352);
#5917=AXIS2_PLACEMENT_3D('',#9050,#7354,#7355);
#5918=AXIS2_PLACEMENT_3D('',#9051,#7356,#7357);
#5919=AXIS2_PLACEMENT_3D('',#9053,#7359,#7360);
#5920=AXIS2_PLACEMENT_3D('',#9054,#7361,#7362);
#5921=AXIS2_PLACEMENT_3D('',#9056,#7364,#7365);
#5922=AXIS2_PLACEMENT_3D('',#9057,#7366,#7367);
#5923=AXIS2_PLACEMENT_3D('',#9059,#7369,#7370);
#5924=AXIS2_PLACEMENT_3D('',#9060,#7371,#7372);
#5925=AXIS2_PLACEMENT_3D('',#9062,#7374,#7375);
#5926=AXIS2_PLACEMENT_3D('',#9063,#7376,#7377);
#5927=AXIS2_PLACEMENT_3D('',#9065,#7379,#7380);
#5928=AXIS2_PLACEMENT_3D('',#9066,#7381,#7382);
#5929=AXIS2_PLACEMENT_3D('',#9068,#7384,#7385);
#5930=AXIS2_PLACEMENT_3D('',#9069,#7386,#7387);
#5931=AXIS2_PLACEMENT_3D('',#9071,#7389,#7390);
#5932=AXIS2_PLACEMENT_3D('',#9073,#7392,#7393);
#5933=AXIS2_PLACEMENT_3D('',#9074,#7394,#7395);
#5934=AXIS2_PLACEMENT_3D('',#9076,#7397,#7398);
#5935=AXIS2_PLACEMENT_3D('',#9078,#7400,#7401);
#5936=AXIS2_PLACEMENT_3D('',#9079,#7402,#7403);
#5937=AXIS2_PLACEMENT_3D('',#9081,#7405,#7406);
#5938=AXIS2_PLACEMENT_3D('',#9083,#7408,#7409);
#5939=AXIS2_PLACEMENT_3D('',#9084,#7410,#7411);
#5940=AXIS2_PLACEMENT_3D('',#9086,#7413,#7414);
#5941=AXIS2_PLACEMENT_3D('',#9088,#7416,#7417);
#5942=AXIS2_PLACEMENT_3D('',#9089,#7418,#7419);
#5943=AXIS2_PLACEMENT_3D('',#9091,#7421,#7422);
#5944=AXIS2_PLACEMENT_3D('',#9093,#7424,#7425);
#5945=AXIS2_PLACEMENT_3D('',#9095,#7427,#7428);
#5946=AXIS2_PLACEMENT_3D('',#9097,#7430,#7431);
#5947=AXIS2_PLACEMENT_3D('',#9098,#7432,#7433);
#5948=AXIS2_PLACEMENT_3D('',#9100,#7435,#7436);
#5949=AXIS2_PLACEMENT_3D('',#9102,#7438,#7439);
#5950=AXIS2_PLACEMENT_3D('',#9104,#7441,#7442);
#5951=AXIS2_PLACEMENT_3D('',#9106,#7444,#7445);
#5952=AXIS2_PLACEMENT_3D('',#9107,#7446,#7447);
#5953=AXIS2_PLACEMENT_3D('',#9109,#7449,#7450);
#5954=AXIS2_PLACEMENT_3D('',#9111,#7452,#7453);
#5955=AXIS2_PLACEMENT_3D('',#9113,#7455,#7456);
#5956=AXIS2_PLACEMENT_3D('',#9115,#7458,#7459);
#5957=AXIS2_PLACEMENT_3D('',#9116,#7460,#7461);
#5958=AXIS2_PLACEMENT_3D('',#9118,#7463,#7464);
#5959=AXIS2_PLACEMENT_3D('',#9120,#7466,#7467);
#5960=AXIS2_PLACEMENT_3D('',#9122,#7469,#7470);
#5961=AXIS2_PLACEMENT_3D('',#9124,#7472,#7473);
#5962=AXIS2_PLACEMENT_3D('',#9125,#7474,#7475);
#5963=AXIS2_PLACEMENT_3D('',#9127,#7477,#7478);
#5964=AXIS2_PLACEMENT_3D('',#9129,#7480,#7481);
#5965=AXIS2_PLACEMENT_3D('',#9131,#7483,#7484);
#5966=AXIS2_PLACEMENT_3D('',#9133,#7486,#7487);
#5967=AXIS2_PLACEMENT_3D('',#9134,#7488,#7489);
#5968=AXIS2_PLACEMENT_3D('',#9136,#7491,#7492);
#5969=AXIS2_PLACEMENT_3D('',#9138,#7494,#7495);
#5970=AXIS2_PLACEMENT_3D('',#9140,#7497,#7498);
#5971=AXIS2_PLACEMENT_3D('',#9142,#7500,#7501);
#5972=AXIS2_PLACEMENT_3D('',#9143,#7502,#7503);
#5973=AXIS2_PLACEMENT_3D('',#9145,#7505,#7506);
#5974=AXIS2_PLACEMENT_3D('',#9147,#7508,#7509);
#5975=AXIS2_PLACEMENT_3D('',#9149,#7511,#7512);
#5976=AXIS2_PLACEMENT_3D('',#9151,#7514,#7515);
#5977=AXIS2_PLACEMENT_3D('',#9152,#7516,#7517);
#5978=AXIS2_PLACEMENT_3D('',#9154,#7519,#7520);
#5979=AXIS2_PLACEMENT_3D('',#9156,#7522,#7523);
#5980=AXIS2_PLACEMENT_3D('',#9158,#7525,#7526);
#5981=AXIS2_PLACEMENT_3D('',#9160,#7528,#7529);
#5982=AXIS2_PLACEMENT_3D('',#9161,#7530,#7531);
#5983=AXIS2_PLACEMENT_3D('',#9163,#7533,#7534);
#5984=AXIS2_PLACEMENT_3D('',#9165,#7536,#7537);
#5985=AXIS2_PLACEMENT_3D('',#9167,#7539,#7540);
#5986=AXIS2_PLACEMENT_3D('',#9169,#7542,#7543);
#5987=AXIS2_PLACEMENT_3D('',#9170,#7544,#7545);
#5988=AXIS2_PLACEMENT_3D('',#9172,#7547,#7548);
#5989=AXIS2_PLACEMENT_3D('',#9174,#7550,#7551);
#5990=AXIS2_PLACEMENT_3D('',#9176,#7553,#7554);
#5991=AXIS2_PLACEMENT_3D('',#9178,#7556,#7557);
#5992=AXIS2_PLACEMENT_3D('',#9179,#7558,#7559);
#5993=AXIS2_PLACEMENT_3D('',#9181,#7561,#7562);
#5994=AXIS2_PLACEMENT_3D('',#9183,#7564,#7565);
#5995=AXIS2_PLACEMENT_3D('',#9185,#7567,#7568);
#5996=AXIS2_PLACEMENT_3D('',#9187,#7570,#7571);
#5997=AXIS2_PLACEMENT_3D('',#9188,#7572,#7573);
#5998=AXIS2_PLACEMENT_3D('',#9190,#7575,#7576);
#5999=AXIS2_PLACEMENT_3D('',#9192,#7578,#7579);
#6000=AXIS2_PLACEMENT_3D('',#9194,#7581,#7582);
#6001=AXIS2_PLACEMENT_3D('',#9196,#7584,#7585);
#6002=AXIS2_PLACEMENT_3D('',#9197,#7586,#7587);
#6003=AXIS2_PLACEMENT_3D('',#9199,#7589,#7590);
#6004=AXIS2_PLACEMENT_3D('',#9201,#7592,#7593);
#6005=AXIS2_PLACEMENT_3D('',#9203,#7595,#7596);
#6006=AXIS2_PLACEMENT_3D('',#9205,#7598,#7599);
#6007=AXIS2_PLACEMENT_3D('',#9206,#7600,#7601);
#6008=AXIS2_PLACEMENT_3D('',#9208,#7603,#7604);
#6009=AXIS2_PLACEMENT_3D('',#9210,#7606,#7607);
#6010=AXIS2_PLACEMENT_3D('',#9212,#7609,#7610);
#6011=AXIS2_PLACEMENT_3D('',#9214,#7612,#7613);
#6012=AXIS2_PLACEMENT_3D('',#9215,#7614,#7615);
#6013=AXIS2_PLACEMENT_3D('',#9218,#7618,#7619);
#6014=AXIS2_PLACEMENT_3D('',#9219,#7620,#7621);
#6334=DIRECTION('axis',(0.,0.,1.));
#6335=DIRECTION('refdir',(1.,0.,0.));
#6336=DIRECTION('center_axis',(0.,0.,1.));
#6337=DIRECTION('ref_axis',(7.80990875742903E-15,-1.,0.));
#6338=DIRECTION('center_axis',(0.,0.,1.));
#6339=DIRECTION('ref_axis',(1.,0.,0.));
#6340=DIRECTION('',(0.,0.,1.));
#6341=DIRECTION('center_axis',(0.,0.,1.));
#6342=DIRECTION('ref_axis',(1.,0.,0.));
#6343=DIRECTION('',(0.,0.,-1.));
#6344=DIRECTION('center_axis',(0.,0.,-1.));
#6345=DIRECTION('ref_axis',(-1.,0.,0.));
#6346=DIRECTION('center_axis',(0.,0.,-1.));
#6347=DIRECTION('ref_axis',(-1.,0.,0.));
#6348=DIRECTION('',(0.,0.,1.));
#6349=DIRECTION('center_axis',(0.,0.,1.));
#6350=DIRECTION('ref_axis',(1.,0.,0.));
#6351=DIRECTION('',(0.,0.,-1.));
#6352=DIRECTION('center_axis',(0.,0.,1.));
#6353=DIRECTION('ref_axis',(1.,0.,0.));
#6354=DIRECTION('center_axis',(1.78945947642876E-15,2.74818654191516E-16,
-1.));
#6355=DIRECTION('ref_axis',(-1.,-3.8094332417834E-33,-1.78945947642876E-15));
#6356=DIRECTION('',(0.,0.,-1.));
#6357=DIRECTION('center_axis',(-8.94729738214379E-16,-1.37409327095758E-16,
-1.));
#6358=DIRECTION('ref_axis',(-1.,-9.5235831044585E-34,8.94729738214379E-16));
#6359=DIRECTION('center_axis',(0.,0.,-1.));
#6360=DIRECTION('ref_axis',(-1.,0.,0.));
#6361=DIRECTION('center_axis',(-1.32139904668388E-15,-6.05000891271787E-16,
-1.));
#6362=DIRECTION('ref_axis',(-1.,1.51602385490383E-31,1.32139904668388E-15));
#6363=DIRECTION('',(0.,0.,1.));
#6364=DIRECTION('center_axis',(0.,0.,1.));
#6365=DIRECTION('ref_axis',(1.,0.,0.));
#6366=DIRECTION('',(0.,0.,-1.));
#6367=DIRECTION('center_axis',(0.,0.,1.));
#6368=DIRECTION('ref_axis',(1.,0.,0.));
#6369=DIRECTION('center_axis',(9.03746752270192E-16,-5.16181690799186E-17,
-1.));
#6370=DIRECTION('ref_axis',(-1.,-1.07685893901274E-34,-9.03746752270192E-16));
#6371=DIRECTION('',(0.,0.,-1.));
#6372=DIRECTION('center_axis',(-9.03746752270196E-16,5.16181690799174E-17,
-1.));
#6373=DIRECTION('ref_axis',(-1.,-1.07685893901823E-34,9.03746752270196E-16));
#6374=DIRECTION('center_axis',(0.,0.,-1.));
#6375=DIRECTION('ref_axis',(-1.,0.,0.));
#6376=DIRECTION('center_axis',(0.,0.,-1.));
#6377=DIRECTION('ref_axis',(-1.,0.,0.));
#6378=DIRECTION('',(0.,0.,1.));
#6379=DIRECTION('center_axis',(0.,0.,1.));
#6380=DIRECTION('ref_axis',(1.,0.,0.));
#6381=DIRECTION('',(0.,0.,-1.));
#6382=DIRECTION('center_axis',(0.,0.,1.));
#6383=DIRECTION('ref_axis',(1.,0.,0.));
#6384=DIRECTION('center_axis',(8.94729738214375E-16,-1.37409327095777E-16,
-1.));
#6385=DIRECTION('ref_axis',(-1.,9.52358310447069E-34,-8.94729738214375E-16));
#6386=DIRECTION('center_axis',(-8.94729738214377E-16,1.37409327095776E-16,
-1.));
#6387=DIRECTION('ref_axis',(-1.,9.52358310446614E-34,8.94729738214377E-16));
#6388=DIRECTION('',(0.,0.,1.));
#6389=DIRECTION('center_axis',(0.,0.,-1.));
#6390=DIRECTION('ref_axis',(-1.,0.,0.));
#6391=DIRECTION('center_axis',(0.,0.,-1.));
#6392=DIRECTION('ref_axis',(-1.,0.,0.));
#6393=DIRECTION('',(0.,0.,1.));
#6394=DIRECTION('center_axis',(0.,0.,1.));
#6395=DIRECTION('ref_axis',(1.,0.,0.));
#6396=DIRECTION('',(0.,0.,-1.));
#6397=DIRECTION('center_axis',(0.,0.,1.));
#6398=DIRECTION('ref_axis',(1.,0.,0.));
#6399=DIRECTION('center_axis',(1.80749350454039E-15,1.03236338159802E-16,
-1.));
#6400=DIRECTION('ref_axis',(-1.,4.30743575605734E-34,-1.80749350454039E-15));
#6401=DIRECTION('center_axis',(-1.80749350454039E-15,-1.03236338159807E-16,
-1.));
#6402=DIRECTION('ref_axis',(-1.,4.30743575606245E-34,1.80749350454039E-15));
#6403=DIRECTION('',(0.,0.,1.));
#6404=DIRECTION('center_axis',(0.,0.,-1.));
#6405=DIRECTION('ref_axis',(-1.,0.,0.));
#6406=DIRECTION('center_axis',(0.,0.,-1.));
#6407=DIRECTION('ref_axis',(-1.,0.,0.));
#6408=DIRECTION('',(0.,0.,1.));
#6409=DIRECTION('center_axis',(0.,0.,1.));
#6410=DIRECTION('ref_axis',(1.,0.,0.));
#6411=DIRECTION('',(0.,0.,-1.));
#6412=DIRECTION('center_axis',(0.,0.,-1.));
#6413=DIRECTION('ref_axis',(-1.,0.,0.));
#6414=DIRECTION('center_axis',(0.,0.,-1.));
#6415=DIRECTION('ref_axis',(-1.,0.,0.));
#6416=DIRECTION('',(0.,0.,1.));
#6417=DIRECTION('center_axis',(0.,0.,1.));
#6418=DIRECTION('ref_axis',(1.,0.,0.));
#6419=DIRECTION('',(0.,0.,-1.));
#6420=DIRECTION('center_axis',(0.,0.,-1.));
#6421=DIRECTION('ref_axis',(-1.,0.,0.));
#6422=DIRECTION('center_axis',(0.,0.,-1.));
#6423=DIRECTION('ref_axis',(-1.,0.,0.));
#6424=DIRECTION('',(0.,0.,1.));
#6425=DIRECTION('center_axis',(0.,0.,1.));
#6426=DIRECTION('ref_axis',(1.,0.,0.));
#6427=DIRECTION('',(0.,0.,-1.));
#6428=DIRECTION('center_axis',(0.,0.,-1.));
#6429=DIRECTION('ref_axis',(-1.,0.,0.));
#6430=DIRECTION('center_axis',(0.,0.,-1.));
#6431=DIRECTION('ref_axis',(-1.,0.,0.));
#6432=DIRECTION('',(0.,0.,1.));
#6433=DIRECTION('center_axis',(0.,0.,1.));
#6434=DIRECTION('ref_axis',(1.,0.,0.));
#6435=DIRECTION('',(0.,0.,-1.));
#6436=DIRECTION('center_axis',(0.,0.,-1.));
#6437=DIRECTION('ref_axis',(-1.,0.,0.));
#6438=DIRECTION('center_axis',(1.18464566449559E-15,8.4186469732886E-16,
-1.));
#6439=DIRECTION('ref_axis',(-1.,9.5828367453829E-32,-1.18464566449559E-15));
#6440=DIRECTION('',(0.,0.,1.));
#6441=DIRECTION('center_axis',(1.18464566449559E-15,8.4186469732886E-16,
1.));
#6442=DIRECTION('ref_axis',(1.,-9.5828367453829E-32,-1.18464566449559E-15));
#6443=DIRECTION('',(0.,0.,-1.));
#6444=DIRECTION('center_axis',(0.,0.,-1.));
#6445=DIRECTION('ref_axis',(-1.,0.,0.));
#6446=DIRECTION('center_axis',(0.,0.,-1.));
#6447=DIRECTION('ref_axis',(-1.,0.,0.));
#6448=DIRECTION('',(0.,0.,1.));
#6449=DIRECTION('center_axis',(0.,0.,1.));
#6450=DIRECTION('ref_axis',(1.,0.,0.));
#6451=DIRECTION('',(0.,0.,-1.));
#6452=DIRECTION('center_axis',(0.,0.,-1.));
#6453=DIRECTION('ref_axis',(-1.,0.,0.));
#6454=DIRECTION('center_axis',(-1.45323412840511E-15,-1.52344036793038E-17,
-1.));
#6455=DIRECTION('ref_axis',(-1.,-2.33073141121972E-33,1.45323412840511E-15));
#6456=DIRECTION('',(0.,0.,1.));
#6457=DIRECTION('center_axis',(0.,0.,1.));
#6458=DIRECTION('ref_axis',(1.,0.,0.));
#6459=DIRECTION('',(0.,0.,-1.));
#6460=DIRECTION('center_axis',(0.,0.,-1.));
#6461=DIRECTION('ref_axis',(-1.,0.,0.));
#6462=DIRECTION('center_axis',(0.,0.,-1.));
#6463=DIRECTION('ref_axis',(-1.,0.,0.));
#6464=DIRECTION('',(0.,0.,1.));
#6465=DIRECTION('center_axis',(0.,0.,1.));
#6466=DIRECTION('ref_axis',(1.,0.,0.));
#6467=DIRECTION('',(0.,0.,-1.));
#6468=DIRECTION('center_axis',(0.,0.,-1.));
#6469=DIRECTION('ref_axis',(-1.,0.,0.));
#6470=DIRECTION('center_axis',(-1.42464488663145E-15,2.87242869383234E-16,
-1.));
#6471=DIRECTION('ref_axis',(-1.,5.21577193803856E-32,1.42464488663145E-15));
#6472=DIRECTION('',(0.,0.,1.));
#6473=DIRECTION('center_axis',(-1.42464488663145E-15,2.87242869383234E-16,
1.));
#6474=DIRECTION('ref_axis',(1.,-5.21577193803856E-32,1.42464488663145E-15));
#6475=DIRECTION('',(0.,0.,-1.));
#6476=DIRECTION('center_axis',(0.,0.,-1.));
#6477=DIRECTION('ref_axis',(-1.,0.,0.));
#6478=DIRECTION('center_axis',(0.,0.,-1.));
#6479=DIRECTION('ref_axis',(-1.,0.,0.));
#6480=DIRECTION('',(0.,0.,1.));
#6481=DIRECTION('center_axis',(0.,0.,1.));
#6482=DIRECTION('ref_axis',(1.,0.,0.));
#6483=DIRECTION('',(0.,0.,-1.));
#6484=DIRECTION('center_axis',(0.,0.,-1.));
#6485=DIRECTION('ref_axis',(-1.,0.,0.));
#6486=DIRECTION('center_axis',(-5.29913193257237E-14,0.,1.));
#6487=DIRECTION('ref_axis',(1.,0.,5.29913193257237E-14));
#6488=DIRECTION('',(0.,0.,-1.));
#6489=DIRECTION('center_axis',(5.29913193257013E-14,0.,1.));
#6490=DIRECTION('ref_axis',(1.,0.,-5.29913193257013E-14));
#6491=DIRECTION('',(0.,0.,1.));
#6492=DIRECTION('center_axis',(0.,0.,-1.));
#6493=DIRECTION('ref_axis',(-1.,0.,0.));
#6494=DIRECTION('center_axis',(-3.54581136321782E-14,-3.93802247521328E-14,
1.));
#6495=DIRECTION('ref_axis',(-8.56410064059132E-32,-1.,-3.93802247521328E-14));
#6496=DIRECTION('',(0.,0.,-1.));
#6497=DIRECTION('center_axis',(3.54581136321784E-14,3.93802247521327E-14,
1.));
#6498=DIRECTION('ref_axis',(-8.56410063443906E-32,-1.,3.93802247521327E-14));
#6499=DIRECTION('',(0.,0.,1.));
#6500=DIRECTION('center_axis',(0.,0.,-1.));
#6501=DIRECTION('ref_axis',(-1.,0.,0.));
#6502=DIRECTION('center_axis',(4.28708778888507E-14,3.11475159991745E-14,
1.));
#6503=DIRECTION('ref_axis',(1.,-1.47528330080296E-31,-4.28708778888507E-14));
#6504=DIRECTION('',(0.,0.,1.));
#6505=DIRECTION('center_axis',(-4.28708778888507E-14,-3.11475159991745E-14,
1.));
#6506=DIRECTION('ref_axis',(1.,-1.47528330080296E-31,4.28708778888507E-14));
#6507=DIRECTION('',(0.,0.,-1.));
#6508=DIRECTION('center_axis',(0.,0.,-1.));
#6509=DIRECTION('ref_axis',(-1.,0.,0.));
#6510=DIRECTION('center_axis',(-2.64956596628557E-14,-4.58918287161186E-14,
1.));
#6511=DIRECTION('ref_axis',(1.05337643511338E-31,-1.,-4.58918287161186E-14));
#6512=DIRECTION('',(0.,0.,-1.));
#6513=DIRECTION('center_axis',(2.64956596628557E-14,4.58918287161186E-14,
1.));
#6514=DIRECTION('ref_axis',(1.05337643511338E-31,-1.,4.58918287161186E-14));
#6515=DIRECTION('',(0.,0.,1.));
#6516=DIRECTION('center_axis',(0.,0.,-1.));
#6517=DIRECTION('ref_axis',(-1.,0.,0.));
#6518=DIRECTION('center_axis',(-1.63752182259927E-14,-5.03977395517881E-14,
1.));
#6519=DIRECTION('ref_axis',(3.95682458153076E-32,-1.,-5.03977395517881E-14));
#6520=DIRECTION('',(0.,0.,-1.));
#6521=DIRECTION('center_axis',(1.63752182259958E-14,5.03977395517984E-14,
1.));
#6522=DIRECTION('ref_axis',(3.95682460883029E-32,-1.,5.03977395517984E-14));
#6523=DIRECTION('',(0.,0.,1.));
#6524=DIRECTION('center_axis',(0.,0.,-1.));
#6525=DIRECTION('ref_axis',(-1.,0.,0.));
#6526=DIRECTION('center_axis',(4.84099790645001E-14,2.1553511334701E-14,
1.));
#6527=DIRECTION('ref_axis',(1.,-5.08629423737342E-32,-4.84099790645001E-14));
#6528=DIRECTION('',(0.,0.,1.));
#6529=DIRECTION('center_axis',(-4.84099790645117E-14,-2.1553511334706E-14,
1.));
#6530=DIRECTION('ref_axis',(1.,-5.08629429118651E-32,4.84099790645117E-14));
#6531=DIRECTION('',(0.,0.,-1.));
#6532=DIRECTION('center_axis',(0.,0.,-1.));
#6533=DIRECTION('ref_axis',(-1.,0.,0.));
#6534=DIRECTION('center_axis',(5.18333318581752E-14,1.1017514799675E-14,
1.));
#6535=DIRECTION('ref_axis',(1.,-2.69341656657878E-32,-5.18333318581752E-14));
#6536=DIRECTION('',(0.,0.,1.));
#6537=DIRECTION('center_axis',(-5.18333318581731E-14,-1.10175147996738E-14,
1.));
#6538=DIRECTION('ref_axis',(1.,-2.69341656387513E-32,5.18333318581731E-14));
#6539=DIRECTION('',(0.,0.,-1.));
#6540=DIRECTION('center_axis',(0.,0.,-1.));
#6541=DIRECTION('ref_axis',(-1.,0.,0.));
#6542=DIRECTION('center_axis',(5.18333318581723E-14,-1.10175147996744E-14,
1.));
#6543=DIRECTION('ref_axis',(1.,2.6934165598586E-32,-5.18333318581723E-14));
#6544=DIRECTION('',(0.,0.,1.));
#6545=DIRECTION('center_axis',(-5.18333318581729E-14,1.10175147996745E-14,
1.));
#6546=DIRECTION('ref_axis',(1.,2.69341656220821E-32,5.18333318581729E-14));
#6547=DIRECTION('',(0.,0.,-1.));
#6548=DIRECTION('center_axis',(0.,0.,-1.));
#6549=DIRECTION('ref_axis',(-1.,0.,0.));
#6550=DIRECTION('center_axis',(-2.64956596628442E-14,4.58918287160994E-14,
1.));
#6551=DIRECTION('ref_axis',(-1.053376425146E-31,-1.,4.58918287160994E-14));
#6552=DIRECTION('',(0.,0.,-1.));
#6553=DIRECTION('center_axis',(2.64956596628505E-14,-4.58918287161103E-14,
1.));
#6554=DIRECTION('ref_axis',(-1.05337643066151E-31,-1.,-4.58918287161103E-14));
#6555=DIRECTION('',(0.,0.,1.));
#6556=DIRECTION('center_axis',(0.,0.,-1.));
#6557=DIRECTION('ref_axis',(-1.,0.,0.));
#6558=DIRECTION('center_axis',(-3.54581136321834E-14,3.93802247521383E-14,
1.));
#6559=DIRECTION('ref_axis',(8.56410059928329E-32,-1.,3.93802247521383E-14));
#6560=DIRECTION('',(0.,0.,-1.));
#6561=DIRECTION('center_axis',(3.54581136321726E-14,-3.93802247521266E-14,
1.));
#6562=DIRECTION('ref_axis',(8.56410068268857E-32,-1.,-3.93802247521266E-14));
#6563=DIRECTION('',(0.,0.,1.));
#6564=DIRECTION('center_axis',(0.,0.,-1.));
#6565=DIRECTION('ref_axis',(-1.,0.,0.));
#6566=DIRECTION('center_axis',(4.8409979064475E-14,-2.15535113346903E-14,
1.));
#6567=DIRECTION('ref_axis',(1.,5.08629413077073E-32,-4.8409979064475E-14));
#6568=DIRECTION('',(0.,0.,1.));
#6569=DIRECTION('center_axis',(-4.84099790644917E-14,2.15535113346974E-14,
1.));
#6570=DIRECTION('ref_axis',(1.,5.08629420584556E-32,4.84099790644917E-14));
#6571=DIRECTION('',(0.,0.,-1.));
#6572=DIRECTION('center_axis',(0.,0.,-1.));
#6573=DIRECTION('ref_axis',(-1.,0.,0.));
#6574=DIRECTION('center_axis',(4.28708778888503E-14,-3.11475159991748E-14,
1.));
#6575=DIRECTION('ref_axis',(1.,1.47528330034113E-31,-4.28708778888503E-14));
#6576=DIRECTION('',(0.,0.,1.));
#6577=DIRECTION('center_axis',(-4.28708778888425E-14,3.11475159991688E-14,
1.));
#6578=DIRECTION('ref_axis',(1.,1.47528329562607E-31,4.28708778888425E-14));
#6579=DIRECTION('',(0.,0.,-1.));
#6580=DIRECTION('center_axis',(0.,0.,-1.));
#6581=DIRECTION('ref_axis',(-1.,0.,0.));
#6582=DIRECTION('center_axis',(1.63752182259953E-14,-5.03977395517968E-14,
1.));
#6583=DIRECTION('ref_axis',(-3.95682460334169E-32,-1.,-5.03977395517968E-14));
#6584=DIRECTION('',(0.,0.,1.));
#6585=DIRECTION('center_axis',(-1.63752182259922E-14,5.03977395517884E-14,
1.));
#6586=DIRECTION('ref_axis',(-3.95682457625739E-32,-1.,5.03977395517884E-14));
#6587=DIRECTION('',(0.,0.,-1.));
#6588=DIRECTION('center_axis',(0.,0.,-1.));
#6589=DIRECTION('ref_axis',(-1.,0.,0.));
#6590=DIRECTION('center_axis',(5.53910117564604E-15,-5.27010273339078E-14,
1.));
#6591=DIRECTION('ref_axis',(1.79740491271749E-32,-1.,-5.27010273339078E-14));
#6592=DIRECTION('',(0.,0.,1.));
#6593=DIRECTION('center_axis',(-5.53910117564605E-15,5.27010273339078E-14,
1.));
#6594=DIRECTION('ref_axis',(1.79740491281615E-32,-1.,5.27010273339078E-14));
#6595=DIRECTION('',(0.,0.,-1.));
#6596=DIRECTION('center_axis',(0.,0.,-1.));
#6597=DIRECTION('ref_axis',(-1.,0.,0.));
#6598=DIRECTION('center_axis',(-5.53910117564048E-15,-5.27010273338518E-14,
1.));
#6599=DIRECTION('ref_axis',(-1.79740495843794E-32,-1.,-5.27010273338518E-14));
#6600=DIRECTION('',(0.,0.,1.));
#6601=DIRECTION('center_axis',(5.53910117564134E-15,5.2701027333863E-14,
1.));
#6602=DIRECTION('ref_axis',(-1.79740494549667E-32,-1.,5.2701027333863E-14));
#6603=DIRECTION('center_axis',(0.,0.,-1.));
#6604=DIRECTION('ref_axis',(-1.,0.,0.));
#6605=DIRECTION('center_axis',(-1.63752182259957E-14,-5.03977395517976E-14,
1.));
#6606=DIRECTION('ref_axis',(3.95682460513535E-32,-1.,-5.03977395517976E-14));
#6607=DIRECTION('',(0.,0.,1.));
#6608=DIRECTION('center_axis',(1.63752182259922E-14,5.03977395517865E-14,
1.));
#6609=DIRECTION('ref_axis',(3.956824570141E-32,-1.,5.03977395517865E-14));
#6610=DIRECTION('center_axis',(0.,0.,-1.));
#6611=DIRECTION('ref_axis',(-1.,0.,0.));
#6612=DIRECTION('center_axis',(1.63752182259915E-14,-5.03977395517886E-14,
1.));
#6613=DIRECTION('ref_axis',(-3.95682457867884E-32,-1.,-5.03977395517886E-14));
#6614=DIRECTION('',(0.,0.,-1.));
#6615=DIRECTION('center_axis',(-1.63752182259948E-14,5.03977395517987E-14,
1.));
#6616=DIRECTION('ref_axis',(-3.95682460886617E-32,-1.,5.03977395517987E-14));
#6617=DIRECTION('center_axis',(0.,0.,-1.));
#6618=DIRECTION('ref_axis',(-1.,0.,0.));
#6619=DIRECTION('center_axis',(2.64956596628546E-14,-4.58918287161192E-14,
1.));
#6620=DIRECTION('ref_axis',(-1.053376435221E-31,-1.,-4.58918287161192E-14));
#6621=DIRECTION('',(0.,0.,-1.));
#6622=DIRECTION('center_axis',(-2.64956596628545E-14,4.58918287161191E-14,
1.));
#6623=DIRECTION('ref_axis',(-1.05337643477796E-31,-1.,4.58918287161191E-14));
#6624=DIRECTION('',(0.,0.,1.));
#6625=DIRECTION('center_axis',(0.,0.,-1.));
#6626=DIRECTION('ref_axis',(-1.,0.,0.));
#6627=DIRECTION('center_axis',(4.28708778888447E-14,-3.11475159991715E-14,
1.));
#6628=DIRECTION('ref_axis',(1.,1.47528329704207E-31,-4.28708778888447E-14));
#6629=DIRECTION('',(0.,0.,-1.));
#6630=DIRECTION('center_axis',(-4.28708778888548E-14,3.11475159991785E-14,
1.));
#6631=DIRECTION('ref_axis',(1.,1.47528330277905E-31,4.28708778888548E-14));
#6632=DIRECTION('',(0.,0.,1.));
#6633=DIRECTION('center_axis',(0.,0.,-1.));
#6634=DIRECTION('ref_axis',(-1.,0.,0.));
#6635=DIRECTION('center_axis',(-3.5458113632178E-14,3.93802247521331E-14,
1.));
#6636=DIRECTION('ref_axis',(8.56410063824163E-32,-1.,3.93802247521331E-14));
#6637=DIRECTION('',(0.,0.,1.));
#6638=DIRECTION('center_axis',(3.54581136321754E-14,-3.93802247521304E-14,
1.));
#6639=DIRECTION('ref_axis',(8.56410065781048E-32,-1.,-3.93802247521304E-14));
#6640=DIRECTION('',(0.,0.,-1.));
#6641=DIRECTION('center_axis',(0.,0.,-1.));
#6642=DIRECTION('ref_axis',(-1.,0.,0.));
#6643=DIRECTION('center_axis',(4.84099790644884E-14,-2.15535113346964E-14,
1.));
#6644=DIRECTION('ref_axis',(1.,5.08629419547381E-32,-4.84099790644884E-14));
#6645=DIRECTION('',(0.,0.,-1.));
#6646=DIRECTION('center_axis',(-4.84099790644954E-14,2.15535113347002E-14,
1.));
#6647=DIRECTION('ref_axis',(1.,5.08629422365244E-32,4.84099790644954E-14));
#6648=DIRECTION('',(0.,0.,1.));
#6649=DIRECTION('center_axis',(0.,0.,-1.));
#6650=DIRECTION('ref_axis',(-1.,0.,0.));
#6651=DIRECTION('center_axis',(5.1833331858162E-14,-1.10175147996729E-14,
1.));
#6652=DIRECTION('ref_axis',(1.,2.6934165387896E-32,-5.1833331858162E-14));
#6653=DIRECTION('',(0.,0.,-1.));
#6654=DIRECTION('center_axis',(-5.18333318581728E-14,1.1017514799675E-14,
1.));
#6655=DIRECTION('ref_axis',(1.,2.69341656191485E-32,5.18333318581728E-14));
#6656=DIRECTION('',(0.,0.,1.));
#6657=DIRECTION('center_axis',(0.,0.,-1.));
#6658=DIRECTION('ref_axis',(1.,-1.00915871466367E-14,0.));
#6659=DIRECTION('center_axis',(5.29913193257013E-14,-5.35591413351499E-28,
1.));
#6660=DIRECTION('ref_axis',(1.,-2.18591407531132E-45,-5.29913193257013E-14));
#6661=DIRECTION('',(0.,0.,-1.));
#6662=DIRECTION('center_axis',(-5.29913193257013E-14,5.35591413351499E-28,
1.));
#6663=DIRECTION('ref_axis',(1.,-2.18591407531132E-45,5.29913193257013E-14));
#6664=DIRECTION('',(0.,0.,1.));
#6665=DIRECTION('center_axis',(0.,0.,-1.));
#6666=DIRECTION('ref_axis',(-1.,0.,0.));
#6667=DIRECTION('center_axis',(5.18333318581513E-14,1.10175147996694E-14,
1.));
#6668=DIRECTION('ref_axis',(1.,-2.69341651343199E-32,-5.18333318581513E-14));
#6669=DIRECTION('',(0.,0.,-1.));
#6670=DIRECTION('center_axis',(-5.18333318581518E-14,-1.10175147996696E-14,
1.));
#6671=DIRECTION('ref_axis',(1.,-2.69341651413071E-32,5.18333318581518E-14));
#6672=DIRECTION('',(0.,0.,1.));
#6673=DIRECTION('center_axis',(0.,0.,-1.));
#6674=DIRECTION('ref_axis',(-1.,0.,0.));
#6675=DIRECTION('center_axis',(3.54581136321655E-14,3.93802247521174E-14,
1.));
#6676=DIRECTION('ref_axis',(-8.56410074679405E-32,-1.,3.93802247521174E-14));
#6677=DIRECTION('',(0.,0.,-1.));
#6678=DIRECTION('center_axis',(-3.54581136321788E-14,-3.93802247521323E-14,
1.));
#6679=DIRECTION('ref_axis',(-8.56410064023259E-32,-1.,-3.93802247521323E-14));
#6680=DIRECTION('',(0.,0.,1.));
#6681=DIRECTION('center_axis',(0.,0.,-1.));
#6682=DIRECTION('ref_axis',(-1.,0.,0.));
#6683=DIRECTION('center_axis',(-2.64956596628558E-14,-4.58918287161185E-14,
1.));
#6684=DIRECTION('ref_axis',(1.05337643492684E-31,-1.,-4.58918287161185E-14));
#6685=DIRECTION('',(0.,0.,1.));
#6686=DIRECTION('center_axis',(2.64956596628559E-14,4.58918287161184E-14,
1.));
#6687=DIRECTION('ref_axis',(1.05337643521562E-31,-1.,4.58918287161184E-14));
#6688=DIRECTION('',(0.,0.,-1.));
#6689=DIRECTION('center_axis',(0.,0.,-1.));
#6690=DIRECTION('ref_axis',(-1.,0.,0.));
#6691=DIRECTION('center_axis',(-4.28708778888579E-14,-3.114751599918E-14,
1.));
#6692=DIRECTION('ref_axis',(1.,-1.47528330530812E-31,4.28708778888579E-14));
#6693=DIRECTION('',(0.,0.,1.));
#6694=DIRECTION('center_axis',(4.28708778888557E-14,3.11475159991785E-14,
1.));
#6695=DIRECTION('ref_axis',(1.,-1.47528330426136E-31,-4.28708778888557E-14));
#6696=DIRECTION('',(0.,0.,-1.));
#6697=DIRECTION('center_axis',(0.,0.,-1.));
#6698=DIRECTION('ref_axis',(-1.,0.,0.));
#6699=DIRECTION('center_axis',(-4.8409979064494E-14,-2.15535113346981E-14,
1.));
#6700=DIRECTION('ref_axis',(1.,-5.0862942118997E-32,4.8409979064494E-14));
#6701=DIRECTION('',(0.,0.,1.));
#6702=DIRECTION('center_axis',(4.84099790644959E-14,2.15535113346995E-14,
1.));
#6703=DIRECTION('ref_axis',(1.,-5.08629422237696E-32,-4.84099790644959E-14));
#6704=DIRECTION('',(0.,0.,-1.));
#6705=DIRECTION('center_axis',(0.,0.,-1.));
#6706=DIRECTION('ref_axis',(-1.,0.,0.));
#6707=DIRECTION('center_axis',(-5.53910117564113E-15,-5.27010273338631E-14,
1.));
#6708=DIRECTION('ref_axis',(-1.7974049544022E-32,-1.,-5.27010273338631E-14));
#6709=DIRECTION('',(0.,0.,-1.));
#6710=DIRECTION('center_axis',(5.53910117564113E-15,5.27010273338631E-14,
1.));
#6711=DIRECTION('ref_axis',(-1.7974049544022E-32,-1.,5.27010273338631E-14));
#6712=DIRECTION('',(0.,0.,1.));
#6713=DIRECTION('center_axis',(0.,0.,1.));
#6714=DIRECTION('ref_axis',(1.,0.,0.));
#6715=DIRECTION('center_axis',(-1.60923747916482E-15,8.29484928207641E-16,
-1.));
#6716=DIRECTION('ref_axis',(-1.,-1.60052481612529E-33,1.60923747916482E-15));
#6717=DIRECTION('center_axis',(0.,0.,1.));
#6718=DIRECTION('ref_axis',(1.,0.,0.));
#6719=DIRECTION('center_axis',(0.,0.,-1.));
#6720=DIRECTION('ref_axis',(-1.,0.,0.));
#6721=DIRECTION('center_axis',(0.,0.,1.));
#6722=DIRECTION('ref_axis',(1.,0.,0.));
#6723=DIRECTION('center_axis',(0.,0.,-1.));
#6724=DIRECTION('ref_axis',(-1.,0.,0.));
#6725=DIRECTION('center_axis',(-7.00806082662238E-16,5.72968988795807E-16,
-1.));
#6726=DIRECTION('ref_axis',(-1.,2.77391763959705E-33,7.00806082662238E-16));
#6727=DIRECTION('center_axis',(0.,0.,1.));
#6728=DIRECTION('ref_axis',(1.,0.,0.));
#6729=DIRECTION('center_axis',(0.,0.,-1.));
#6730=DIRECTION('ref_axis',(-1.,0.,0.));
#6731=DIRECTION('center_axis',(4.63562821373925E-16,1.3774000978861E-15,
1.));
#6732=DIRECTION('ref_axis',(-1.06074921525595E-31,-1.,1.3774000978861E-15));
#6733=DIRECTION('center_axis',(2.9160531709346E-16,-1.78680073022012E-15,
-1.));
#6734=DIRECTION('ref_axis',(-4.81742820615547E-33,1.,-1.78680073022012E-15));
#6735=DIRECTION('center_axis',(-5.66364837089041E-16,7.06154019267167E-16,
-1.));
#6736=DIRECTION('ref_axis',(2.86938317203061E-34,1.,7.06154019267168E-16));
#6737=DIRECTION('center_axis',(0.,0.,1.));
#6738=DIRECTION('ref_axis',(1.,0.,0.));
#6739=DIRECTION('center_axis',(0.,0.,-1.));
#6740=DIRECTION('ref_axis',(-1.,0.,0.));
#6741=DIRECTION('center_axis',(0.,0.,1.));
#6742=DIRECTION('ref_axis',(1.,0.,0.));
#6743=DIRECTION('center_axis',(-4.31318598491438E-17,-9.04191500891283E-16,
-1.));
#6744=DIRECTION('ref_axis',(-1.09164579339903E-34,1.,-9.04191500891283E-16));
#6745=DIRECTION('center_axis',(0.,0.,-1.));
#6746=DIRECTION('ref_axis',(-1.,0.,0.));
#6747=DIRECTION('center_axis',(1.18464566449553E-15,-8.41864697328891E-16,
1.));
#6748=DIRECTION('ref_axis',(1.,9.58283674537864E-32,-1.18464566449553E-15));
#6749=DIRECTION('center_axis',(0.,0.,-1.));
#6750=DIRECTION('ref_axis',(-1.,0.,0.));
#6751=DIRECTION('center_axis',(9.83724801784613E-16,1.06976961695994E-15,
1.));
#6752=DIRECTION('ref_axis',(-1.03029779618179E-33,-1.,1.06976961695994E-15));
#6753=DIRECTION('center_axis',(-2.3018130899998E-16,-8.75465129291354E-16,
-1.));
#6754=DIRECTION('ref_axis',(-2.99401685848927E-33,1.,-8.75465129291354E-16));
#6755=DIRECTION('center_axis',(0.,0.,-1.));
#6756=DIRECTION('ref_axis',(-1.,0.,0.));
#6757=DIRECTION('center_axis',(0.,0.,1.));
#6758=DIRECTION('ref_axis',(1.,0.,0.));
#6759=DIRECTION('center_axis',(0.,0.,-1.));
#6760=DIRECTION('ref_axis',(-1.,0.,0.));
#6761=DIRECTION('center_axis',(0.,0.,1.));
#6762=DIRECTION('ref_axis',(1.,0.,0.));
#6763=DIRECTION('center_axis',(-8.14341460830106E-16,-1.61695346118725E-15,
-1.));
#6764=DIRECTION('ref_axis',(-7.85474895342403E-33,1.,-1.61695346118725E-15));
#6765=DIRECTION('center_axis',(-8.62637196982729E-17,1.80838300178258E-15,
-1.));
#6766=DIRECTION('ref_axis',(4.36658317362438E-34,1.,1.80838300178258E-15));
#6767=DIRECTION('center_axis',(0.,0.,1.));
#6768=DIRECTION('ref_axis',(1.,0.,0.));
#6769=DIRECTION('center_axis',(0.,0.,-1.));
#6770=DIRECTION('ref_axis',(-1.,0.,0.));
#6771=DIRECTION('center_axis',(0.,0.,1.));
#6772=DIRECTION('ref_axis',(1.,0.,0.));
#6773=DIRECTION('center_axis',(-1.1327296741781E-15,-1.41230803853433E-15,
-1.));
#6774=DIRECTION('ref_axis',(-1.14775326881119E-33,1.,-1.41230803853433E-15));
#6775=DIRECTION('center_axis',(2.91605317093473E-16,1.78680073022013E-15,
-1.));
#6776=DIRECTION('ref_axis',(4.81742820615223E-33,1.,1.78680073022013E-15));
#6777=DIRECTION('center_axis',(0.,0.,1.));
#6778=DIRECTION('ref_axis',(1.,0.,0.));
#6779=DIRECTION('center_axis',(0.,0.,-1.));
#6780=DIRECTION('ref_axis',(-1.,0.,0.));
#6781=DIRECTION('center_axis',(0.,0.,1.));
#6782=DIRECTION('ref_axis',(1.,0.,0.));
#6783=DIRECTION('center_axis',(-7.00806082662235E-16,-5.72968988795798E-16,
-1.));
#6784=DIRECTION('ref_axis',(-1.,-2.77391763959813E-33,7.00806082662235E-16));
#6785=DIRECTION('center_axis',(6.5672980225067E-16,1.68712669272586E-15,
-1.));
#6786=DIRECTION('ref_axis',(-9.28280238043588E-34,1.,1.68712669272585E-15));
#6787=DIRECTION('center_axis',(0.,0.,1.));
#6788=DIRECTION('ref_axis',(1.,0.,0.));
#6789=DIRECTION('center_axis',(0.,0.,-1.));
#6790=DIRECTION('ref_axis',(-1.,0.,0.));
#6791=DIRECTION('center_axis',(1.45323412840514E-15,-1.52344036793355E-17,
1.));
#6792=DIRECTION('ref_axis',(1.,-2.33073141122416E-33,-1.45323412840514E-15));
#6793=DIRECTION('center_axis',(-8.04618739582399E-16,-4.14742464103809E-16,
-1.));
#6794=DIRECTION('ref_axis',(-1.,-7.72936702803813E-33,8.04618739582399E-16));
#6795=DIRECTION('center_axis',(9.93152043710288E-16,1.51371712302743E-15,
-1.));
#6796=DIRECTION('ref_axis',(1.50815602913674E-32,1.,1.51371712302743E-15));
#6797=DIRECTION('center_axis',(1.3675338218833E-16,1.44686558860067E-15,
1.));
#6798=DIRECTION('ref_axis',(-2.17929987622515E-32,-1.,1.44686558860067E-15));
#6799=DIRECTION('center_axis',(0.,0.,-1.));
#6800=DIRECTION('ref_axis',(-1.,0.,0.));
#6801=DIRECTION('center_axis',(0.,0.,1.));
#6802=DIRECTION('ref_axis',(1.,0.,0.));
#6803=DIRECTION('center_axis',(-8.73265696593734E-16,-2.38389703575337E-16,
-1.));
#6804=DIRECTION('ref_axis',(-1.,2.57646307002847E-33,8.73265696593734E-16));
#6805=DIRECTION('center_axis',(1.28616877518753E-15,1.27415085143204E-15,
-1.));
#6806=DIRECTION('ref_axis',(-1.,-9.57919634854104E-33,-1.28616877518753E-15));
#6807=DIRECTION('center_axis',(0.,0.,1.));
#6808=DIRECTION('ref_axis',(1.,0.,0.));
#6809=DIRECTION('center_axis',(0.,0.,-1.));
#6810=DIRECTION('ref_axis',(-1.,0.,0.));
#6811=DIRECTION('center_axis',(0.,0.,1.));
#6812=DIRECTION('ref_axis',(1.,0.,0.));
#6813=DIRECTION('center_axis',(0.,0.,-1.));
#6814=DIRECTION('ref_axis',(-1.,0.,0.));
#6815=DIRECTION('center_axis',(0.,0.,-1.));
#6816=DIRECTION('ref_axis',(-1.,0.,0.));
#6817=DIRECTION('center_axis',(0.,0.,1.));
#6818=DIRECTION('ref_axis',(1.,0.,0.));
#6819=DIRECTION('center_axis',(0.,0.,-1.));
#6820=DIRECTION('ref_axis',(-1.,0.,0.));
#6821=DIRECTION('center_axis',(0.,0.,1.));
#6822=DIRECTION('ref_axis',(1.,0.,0.));
#6823=DIRECTION('center_axis',(-8.94729738214378E-16,1.37409327095771E-16,
-1.));
#6824=DIRECTION('ref_axis',(-1.,9.52358310446502E-34,8.94729738214378E-16));
#6825=DIRECTION('center_axis',(1.69321748241794E-15,6.40862752628506E-16,
-1.));
#6826=DIRECTION('ref_axis',(-1.,4.80921258843877E-33,-1.69321748241794E-15));
#6827=DIRECTION('center_axis',(0.,0.,1.));
#6828=DIRECTION('ref_axis',(1.,0.,0.));
#6829=DIRECTION('center_axis',(0.,0.,-1.));
#6830=DIRECTION('ref_axis',(-1.,0.,0.));
#6831=DIRECTION('center_axis',(0.,0.,1.));
#6832=DIRECTION('ref_axis',(1.,0.,0.));
#6833=DIRECTION('center_axis',(-1.69321748241794E-15,6.40862752628506E-16,
-1.));
#6834=DIRECTION('ref_axis',(-1.,-4.80921258844117E-33,1.69321748241794E-15));
#6835=DIRECTION('center_axis',(0.,0.,-1.));
#6836=DIRECTION('ref_axis',(-1.,0.,0.));
#6837=DIRECTION('center_axis',(0.,0.,1.));
#6838=DIRECTION('ref_axis',(1.,0.,0.));
#6839=DIRECTION('center_axis',(-7.61486879733257E-16,4.89449036787473E-16,
-1.));
#6840=DIRECTION('ref_axis',(-1.,-8.14289481143214E-33,7.61486879733257E-16));
#6841=DIRECTION('center_axis',(0.,0.,-1.));
#6842=DIRECTION('ref_axis',(-1.,0.,0.));
#6843=DIRECTION('center_axis',(0.,0.,1.));
#6844=DIRECTION('ref_axis',(1.,0.,0.));
#6845=DIRECTION('center_axis',(-6.43084387593755E-16,6.37075425716024E-16,
-1.));
#6846=DIRECTION('ref_axis',(-1.,-1.00927178548204E-32,6.43084387593755E-16));
#6847=DIRECTION('center_axis',(1.74653139318747E-15,-4.76779407150702E-16,
-1.));
#6848=DIRECTION('ref_axis',(-1.,8.38515567293037E-33,-1.74653139318747E-15));
#6849=DIRECTION('center_axis',(0.,0.,-1.));
#6850=DIRECTION('ref_axis',(-1.,0.,0.));
#6851=DIRECTION('center_axis',(0.,0.,1.));
#6852=DIRECTION('ref_axis',(1.,0.,0.));
#6853=DIRECTION('center_axis',(0.,0.,-1.));
#6854=DIRECTION('ref_axis',(-1.,0.,0.));
#6855=DIRECTION('center_axis',(8.04618739582395E-16,-4.14742464103823E-16,
-1.));
#6856=DIRECTION('ref_axis',(-1.,7.72936702804043E-33,-8.04618739582395E-16));
#6857=DIRECTION('center_axis',(0.,0.,-1.));
#6858=DIRECTION('ref_axis',(-1.,0.,0.));
#6859=DIRECTION('center_axis',(0.,0.,1.));
#6860=DIRECTION('ref_axis',(1.,0.,0.));
#6861=DIRECTION('center_axis',(0.,0.,-1.));
#6862=DIRECTION('ref_axis',(-1.,0.,0.));
#6863=DIRECTION('center_axis',(1.40161216532447E-15,-1.14593797759163E-15,
-1.));
#6864=DIRECTION('ref_axis',(-1.,1.10956705583757E-32,-1.40161216532447E-15));
#6865=DIRECTION('center_axis',(0.,0.,-1.));
#6866=DIRECTION('ref_axis',(-1.,0.,0.));
#6867=DIRECTION('center_axis',(0.,0.,1.));
#6868=DIRECTION('ref_axis',(1.,0.,0.));
#6869=DIRECTION('center_axis',(-2.91605317093444E-16,1.78680073022012E-15,
-1.));
#6870=DIRECTION('ref_axis',(-4.81742820615669E-33,1.,1.78680073022012E-15));
#6871=DIRECTION('center_axis',(0.,0.,-1.));
#6872=DIRECTION('ref_axis',(-1.,0.,0.));
#6873=DIRECTION('center_axis',(0.,0.,-1.));
#6874=DIRECTION('ref_axis',(-1.,0.,0.));
#6875=DIRECTION('center_axis',(-7.39810444800344E-16,-1.25092047100568E-15,
1.));
#6876=DIRECTION('ref_axis',(1.33242458232468E-31,-1.,-1.25092047100568E-15));
#6877=DIRECTION('center_axis',(4.31318598491496E-17,9.04191500891285E-16,
-1.));
#6878=DIRECTION('ref_axis',(-1.09164579339958E-34,1.,9.04191500891285E-16));
#6879=DIRECTION('center_axis',(4.07170730415042E-16,-8.08476730593626E-16,
-1.));
#6880=DIRECTION('ref_axis',(-6.01739504654964E-33,1.,-8.08476730593626E-16));
#6881=DIRECTION('center_axis',(0.,0.,-1.));
#6882=DIRECTION('ref_axis',(-1.,0.,0.));
#6883=DIRECTION('center_axis',(0.,0.,1.));
#6884=DIRECTION('ref_axis',(1.,0.,0.));
#6885=DIRECTION('center_axis',(2.30181308999987E-16,8.75465129291357E-16,
-1.));
#6886=DIRECTION('ref_axis',(-2.99401685849059E-33,1.,8.75465129291357E-16));
#6887=DIRECTION('center_axis',(2.3018130899997E-16,-8.75465129291361E-16,
-1.));
#6888=DIRECTION('ref_axis',(2.99401685849076E-33,1.,-8.75465129291361E-16));
#6889=DIRECTION('center_axis',(0.,0.,1.));
#6890=DIRECTION('ref_axis',(1.,0.,0.));
#6891=DIRECTION('center_axis',(0.,0.,-1.));
#6892=DIRECTION('ref_axis',(-1.,0.,0.));
#6893=DIRECTION('center_axis',(0.,0.,-1.));
#6894=DIRECTION('ref_axis',(-1.,0.,0.));
#6895=DIRECTION('center_axis',(8.62637196982607E-17,-1.80838300178258E-15,
-1.));
#6896=DIRECTION('ref_axis',(4.36658317360467E-34,1.,-1.80838300178258E-15));
#6897=DIRECTION('center_axis',(0.,0.,1.));
#6898=DIRECTION('ref_axis',(1.,0.,0.));
#6899=DIRECTION('center_axis',(0.,0.,-1.));
#6900=DIRECTION('ref_axis',(-1.,0.,0.));
#6901=DIRECTION('center_axis',(1.13272967417811E-15,1.41230803853433E-15,
-1.));
#6902=DIRECTION('ref_axis',(-1.1477532688217E-33,1.,1.41230803853433E-15));
#6903=DIRECTION('center_axis',(-1.4580265854674E-16,-8.93400365110051E-16,
-1.));
#6904=DIRECTION('ref_axis',(1.20435705154195E-33,1.,-8.9340036511005E-16));
#6905=DIRECTION('center_axis',(0.,0.,1.));
#6906=DIRECTION('ref_axis',(1.,0.,0.));
#6907=DIRECTION('center_axis',(0.,0.,-1.));
#6908=DIRECTION('ref_axis',(-1.,0.,0.));
#6909=DIRECTION('center_axis',(7.00806082662235E-16,5.7296898879579E-16,
-1.));
#6910=DIRECTION('ref_axis',(-1.,-2.77391763960031E-33,-7.00806082662235E-16));
#6911=DIRECTION('center_axis',(-6.5672980225068E-16,-1.68712669272586E-15,
-1.));
#6912=DIRECTION('ref_axis',(-9.28280238055324E-34,1.,-1.68712669272586E-15));
#6913=DIRECTION('center_axis',(0.,0.,1.));
#6914=DIRECTION('ref_axis',(1.,0.,0.));
#6915=DIRECTION('center_axis',(0.,0.,-1.));
#6916=DIRECTION('ref_axis',(-1.,0.,0.));
#6917=DIRECTION('center_axis',(0.,0.,-1.));
#6918=DIRECTION('ref_axis',(-1.,0.,0.));
#6919=DIRECTION('center_axis',(-9.93152043710293E-16,-1.51371712302739E-15,
-1.));
#6920=DIRECTION('ref_axis',(1.50815602914153E-32,1.,-1.51371712302739E-15));
#6921=DIRECTION('center_axis',(0.,0.,1.));
#6922=DIRECTION('ref_axis',(1.,0.,0.));
#6923=DIRECTION('center_axis',(0.,0.,-1.));
#6924=DIRECTION('ref_axis',(-1.,0.,0.));
#6925=DIRECTION('center_axis',(8.73265696593737E-16,2.38389703575328E-16,
-1.));
#6926=DIRECTION('ref_axis',(-1.,2.57646307002799E-33,-8.73265696593737E-16));
#6927=DIRECTION('center_axis',(-6.43084387593757E-16,-6.37075425716002E-16,
-1.));
#6928=DIRECTION('ref_axis',(-1.,1.00927178548153E-32,6.43084387593757E-16));
#6929=DIRECTION('center_axis',(0.,0.,1.));
#6930=DIRECTION('ref_axis',(1.,0.,0.));
#6931=DIRECTION('center_axis',(0.,0.,-1.));
#6932=DIRECTION('ref_axis',(-1.,0.,0.));
#6933=DIRECTION('center_axis',(-1.52297375946654E-15,-9.78898073574922E-16,
-1.));
#6934=DIRECTION('ref_axis',(-1.,-5.80380233320457E-33,1.52297375946654E-15));
#6935=DIRECTION('center_axis',(0.,0.,1.));
#6936=DIRECTION('ref_axis',(1.,0.,0.));
#6937=DIRECTION('center_axis',(0.,0.,-1.));
#6938=DIRECTION('ref_axis',(-1.,0.,0.));
#6939=DIRECTION('center_axis',(-5.53910117564523E-15,5.27010273339079E-14,
1.));
#6940=DIRECTION('ref_axis',(1.79740492095489E-32,-1.,5.27010273339079E-14));
#6941=DIRECTION('center_axis',(-8.46608741208968E-16,-3.20431376314253E-16,
-1.));
#6942=DIRECTION('ref_axis',(-1.,-5.07857362029075E-33,8.46608741208968E-16));
#6943=DIRECTION('center_axis',(0.,0.,1.));
#6944=DIRECTION('ref_axis',(1.,0.,0.));
#6945=DIRECTION('center_axis',(0.,0.,-1.));
#6946=DIRECTION('ref_axis',(-1.,0.,0.));
#6947=DIRECTION('center_axis',(0.,0.,1.));
#6948=DIRECTION('ref_axis',(1.,0.,0.));
#6949=DIRECTION('center_axis',(8.46608741208968E-16,-3.20431376314254E-16,
-1.));
#6950=DIRECTION('ref_axis',(-1.,5.07857362029218E-33,-8.46608741208968E-16));
#6951=DIRECTION('center_axis',(-8.94729738214377E-16,-1.37409327095765E-16,
-1.));
#6952=DIRECTION('ref_axis',(-1.,-9.52358310446232E-34,8.94729738214377E-16));
#6953=DIRECTION('center_axis',(0.,0.,1.));
#6954=DIRECTION('ref_axis',(1.,0.,0.));
#6955=DIRECTION('center_axis',(0.,0.,-1.));
#6956=DIRECTION('ref_axis',(-1.,0.,0.));
#6957=DIRECTION('center_axis',(0.,0.,1.));
#6958=DIRECTION('ref_axis',(1.,0.,0.));
#6959=DIRECTION('center_axis',(7.61486879733261E-16,-4.89449036787468E-16,
-1.));
#6960=DIRECTION('ref_axis',(-1.,-8.14289481143569E-33,-7.61486879733261E-16));
#6961=DIRECTION('center_axis',(-9.03746752270189E-16,5.16181690799129E-17,
-1.));
#6962=DIRECTION('ref_axis',(-1.,-1.07685893901366E-34,9.03746752270189E-16));
#6963=DIRECTION('center_axis',(0.,0.,1.));
#6964=DIRECTION('ref_axis',(1.,0.,0.));
#6965=DIRECTION('center_axis',(0.,0.,-1.));
#6966=DIRECTION('ref_axis',(-1.,0.,0.));
#6967=DIRECTION('center_axis',(-4.34585263591718E-16,1.38681547715823E-15,
1.));
#6968=DIRECTION('ref_axis',(9.53523368488341E-32,-1.,1.38681547715823E-15));
#6969=DIRECTION('center_axis',(0.,0.,-1.));
#6970=DIRECTION('ref_axis',(-1.,0.,0.));
#6971=DIRECTION('center_axis',(0.,0.,-1.));
#6972=DIRECTION('ref_axis',(-1.,0.,0.));
#6973=DIRECTION('center_axis',(0.,0.,1.));
#6974=DIRECTION('ref_axis',(1.,0.,0.));
#6975=DIRECTION('center_axis',(0.,0.,-1.));
#6976=DIRECTION('ref_axis',(-1.,0.,0.));
#6977=DIRECTION('center_axis',(-1.36753382188316E-16,1.44686558860067E-15,
1.));
#6978=DIRECTION('ref_axis',(2.17929987622488E-32,-1.,1.44686558860067E-15));
#6979=DIRECTION('center_axis',(4.96576021855139E-16,-7.5685856151371E-16,
-1.));
#6980=DIRECTION('ref_axis',(5.96315361064996E-33,1.,-7.5685856151371E-16));
#6981=DIRECTION('',(-1.,0.,0.));
#6982=DIRECTION('',(1.13134139737618E-16,-1.,0.));
#6983=DIRECTION('',(1.13134139737618E-16,1.,0.));
#6984=DIRECTION('center_axis',(0.,0.,1.));
#6985=DIRECTION('ref_axis',(1.,0.,0.));
#6986=DIRECTION('center_axis',(1.60923747916481E-15,-8.29484928207644E-16,
-1.));
#6987=DIRECTION('ref_axis',(-1.,-1.60052481610948E-33,-1.60923747916481E-15));
#6988=DIRECTION('center_axis',(-9.93152043710277E-16,1.51371712302743E-15,
-1.));
#6989=DIRECTION('ref_axis',(-1.50815602913694E-32,1.,1.51371712302743E-15));
#6990=DIRECTION('center_axis',(-1.36753382188316E-16,1.44686558860067E-15,
-1.));
#6991=DIRECTION('ref_axis',(-2.17929987622498E-32,1.,1.44686558860067E-15));
#6992=DIRECTION('center_axis',(0.,0.,-1.));
#6993=DIRECTION('ref_axis',(-1.,0.,0.));
#6994=DIRECTION('center_axis',(0.,0.,-1.));
#6995=DIRECTION('ref_axis',(-1.,0.,0.));
#6996=DIRECTION('center_axis',(8.73265696593735E-16,-2.38389703575344E-16,
-1.));
#6997=DIRECTION('ref_axis',(-1.,-2.57646307002882E-33,-8.73265696593735E-16));
#6998=DIRECTION('center_axis',(0.,0.,-1.));
#6999=DIRECTION('ref_axis',(-1.,0.,0.));
#7000=DIRECTION('center_axis',(-4.34585263591734E-16,1.38681547715824E-15,
-1.));
#7001=DIRECTION('ref_axis',(-9.53523368488213E-32,1.,1.38681547715824E-15));
#7002=DIRECTION('center_axis',(0.,0.,-1.));
#7003=DIRECTION('ref_axis',(-1.,0.,0.));
#7004=DIRECTION('center_axis',(0.,0.,-1.));
#7005=DIRECTION('ref_axis',(-1.,0.,0.));
#7006=DIRECTION('center_axis',(0.,0.,-1.));
#7007=DIRECTION('ref_axis',(-1.,0.,0.));
#7008=DIRECTION('center_axis',(-1.52297375946653E-15,9.78898073574935E-16,
-1.));
#7009=DIRECTION('ref_axis',(-1.,5.80380233323614E-33,1.52297375946653E-15));
#7010=DIRECTION('center_axis',(0.,0.,-1.));
#7011=DIRECTION('ref_axis',(-1.,0.,0.));
#7012=DIRECTION('center_axis',(0.,0.,-1.));
#7013=DIRECTION('ref_axis',(-1.,0.,0.));
#7014=DIRECTION('center_axis',(0.,0.,-1.));
#7015=DIRECTION('ref_axis',(-1.,0.,0.));
#7016=DIRECTION('center_axis',(8.9472973821438E-16,1.37409327095766E-16,
-1.));
#7017=DIRECTION('ref_axis',(-1.,-9.52358310444862E-34,-8.94729738214381E-16));
#7018=DIRECTION('center_axis',(-8.4660874120897E-16,3.20431376314254E-16,
-1.));
#7019=DIRECTION('ref_axis',(-1.,5.07857362028999E-33,8.4660874120897E-16));
#7020=DIRECTION('center_axis',(0.,0.,-1.));
#7021=DIRECTION('ref_axis',(-1.,0.,0.));
#7022=DIRECTION('center_axis',(0.,0.,-1.));
#7023=DIRECTION('ref_axis',(-1.,0.,0.));
#7024=DIRECTION('center_axis',(0.,0.,-1.));
#7025=DIRECTION('ref_axis',(-1.,0.,0.));
#7026=DIRECTION('center_axis',(0.,0.,-1.));
#7027=DIRECTION('ref_axis',(-1.,0.,0.));
#7028=DIRECTION('center_axis',(5.53910117564333E-15,-5.27010273338855E-14,
1.));
#7029=DIRECTION('ref_axis',(1.79740494482853E-32,-1.,-5.27010273338855E-14));
#7030=DIRECTION('center_axis',(0.,0.,-1.));
#7031=DIRECTION('ref_axis',(-1.,0.,0.));
#7032=DIRECTION('center_axis',(0.,0.,-1.));
#7033=DIRECTION('ref_axis',(-1.,0.,0.));
#7034=DIRECTION('center_axis',(7.61486879733267E-16,4.89449036787458E-16,
-1.));
#7035=DIRECTION('ref_axis',(-1.,8.14289481143805E-33,-7.61486879733267E-16));
#7036=DIRECTION('center_axis',(0.,0.,-1.));
#7037=DIRECTION('ref_axis',(-1.,0.,0.));
#7038=DIRECTION('center_axis',(4.34585263591789E-16,1.38681547715822E-15,
-1.));
#7039=DIRECTION('ref_axis',(9.53523368488375E-32,1.,1.38681547715822E-15));
#7040=DIRECTION('center_axis',(6.43084387593757E-16,6.37075425716005E-16,
-1.));
#7041=DIRECTION('ref_axis',(-1.,1.00927178548155E-32,-6.43084387593758E-16));
#7042=DIRECTION('center_axis',(-8.73265696593747E-16,-2.38389703575334E-16,
-1.));
#7043=DIRECTION('ref_axis',(-1.,2.57646307003222E-33,8.73265696593746E-16));
#7044=DIRECTION('center_axis',(0.,0.,-1.));
#7045=DIRECTION('ref_axis',(-1.,0.,0.));
#7046=DIRECTION('center_axis',(0.,0.,-1.));
#7047=DIRECTION('ref_axis',(-1.,0.,0.));
#7048=DIRECTION('center_axis',(4.96576021855147E-16,7.568585615137E-16,
-1.));
#7049=DIRECTION('ref_axis',(-5.96315361064353E-33,1.,7.568585615137E-16));
#7050=DIRECTION('center_axis',(0.,0.,-1.));
#7051=DIRECTION('ref_axis',(-1.,0.,0.));
#7052=DIRECTION('center_axis',(0.,0.,-1.));
#7053=DIRECTION('ref_axis',(-1.,0.,0.));
#7054=DIRECTION('center_axis',(0.,0.,-1.));
#7055=DIRECTION('ref_axis',(-1.,0.,0.));
#7056=DIRECTION('center_axis',(6.56729802250692E-16,1.68712669272589E-15,
-1.));
#7057=DIRECTION('ref_axis',(-9.28280238086152E-34,1.,1.68712669272589E-15));
#7058=DIRECTION('center_axis',(-7.00806082662247E-16,-5.72968988795798E-16,
-1.));
#7059=DIRECTION('ref_axis',(-1.,-2.77391763959015E-33,7.00806082662247E-16));
#7060=DIRECTION('center_axis',(0.,0.,-1.));
#7061=DIRECTION('ref_axis',(-1.,0.,0.));
#7062=DIRECTION('center_axis',(0.,0.,-1.));
#7063=DIRECTION('ref_axis',(-1.,0.,0.));
#7064=DIRECTION('center_axis',(1.45802658546741E-16,8.93400365110057E-16,
-1.));
#7065=DIRECTION('ref_axis',(1.20435705154029E-33,1.,8.93400365110057E-16));
#7066=DIRECTION('center_axis',(-5.66364837089057E-16,-7.06154019267168E-16,
-1.));
#7067=DIRECTION('ref_axis',(-2.8693831720744E-34,1.,-7.06154019267168E-16));
#7068=DIRECTION('center_axis',(0.,0.,-1.));
#7069=DIRECTION('ref_axis',(-1.,0.,0.));
#7070=DIRECTION('center_axis',(0.,0.,-1.));
#7071=DIRECTION('ref_axis',(-1.,0.,0.));
#7072=DIRECTION('center_axis',(-8.62637196982615E-17,1.80838300178258E-15,
-1.));
#7073=DIRECTION('ref_axis',(4.3665831736119E-34,1.,1.80838300178258E-15));
#7074=DIRECTION('center_axis',(-8.14341460830121E-16,-1.61695346118725E-15,
-1.));
#7075=DIRECTION('ref_axis',(-7.85474895342543E-33,1.,-1.61695346118725E-15));
#7076=DIRECTION('center_axis',(0.,0.,-1.));
#7077=DIRECTION('ref_axis',(-1.,0.,0.));
#7078=DIRECTION('center_axis',(0.,0.,-1.));
#7079=DIRECTION('ref_axis',(-1.,0.,0.));
#7080=DIRECTION('center_axis',(-2.3018130899997E-16,8.75465129291364E-16,
-1.));
#7081=DIRECTION('ref_axis',(2.9940168584926E-33,1.,8.75465129291364E-16));
#7082=DIRECTION('center_axis',(-2.30181308999987E-16,-8.75465129291357E-16,
-1.));
#7083=DIRECTION('ref_axis',(-2.99401685849059E-33,1.,-8.75465129291357E-16));
#7084=DIRECTION('center_axis',(0.,0.,-1.));
#7085=DIRECTION('ref_axis',(-1.,0.,0.));
#7086=DIRECTION('center_axis',(0.,0.,-1.));
#7087=DIRECTION('ref_axis',(-1.,0.,0.));
#7088=DIRECTION('center_axis',(-4.07170730415043E-16,8.08476730593629E-16,
-1.));
#7089=DIRECTION('ref_axis',(-6.01739504654846E-33,1.,8.08476730593629E-16));
#7090=DIRECTION('center_axis',(-4.31318598491494E-17,-9.04191500891281E-16,
-1.));
#7091=DIRECTION('ref_axis',(-1.09164579339739E-34,1.,-9.04191500891281E-16));
#7092=DIRECTION('center_axis',(-7.39810444800352E-16,-1.25092047100568E-15,
-1.));
#7093=DIRECTION('ref_axis',(-1.33242458232479E-31,1.,-1.25092047100568E-15));
#7094=DIRECTION('center_axis',(0.,0.,-1.));
#7095=DIRECTION('ref_axis',(-1.,0.,0.));
#7096=DIRECTION('center_axis',(0.,0.,-1.));
#7097=DIRECTION('ref_axis',(-1.,0.,0.));
#7098=DIRECTION('center_axis',(2.91605317093441E-16,-1.78680073022012E-15,
-1.));
#7099=DIRECTION('ref_axis',(-4.81742820615958E-33,1.,-1.78680073022012E-15));
#7100=DIRECTION('center_axis',(-4.63562821373958E-16,-1.37740009788611E-15,
-1.));
#7101=DIRECTION('ref_axis',(1.06074921525593E-31,1.,-1.37740009788611E-15));
#7102=DIRECTION('center_axis',(0.,0.,-1.));
#7103=DIRECTION('ref_axis',(-1.,0.,0.));
#7104=DIRECTION('center_axis',(-1.40161216532447E-15,1.14593797759164E-15,
-1.));
#7105=DIRECTION('ref_axis',(-1.,1.10956705583637E-32,1.40161216532447E-15));
#7106=DIRECTION('center_axis',(3.28364901125325E-16,-8.43563346362936E-16,
-1.));
#7107=DIRECTION('ref_axis',(-6.20431423727392E-33,1.,-8.43563346362936E-16));
#7108=DIRECTION('center_axis',(0.,0.,-1.));
#7109=DIRECTION('ref_axis',(-1.,0.,0.));
#7110=DIRECTION('center_axis',(0.,0.,-1.));
#7111=DIRECTION('ref_axis',(-1.,0.,0.));
#7112=DIRECTION('center_axis',(-1.60923747916479E-15,8.29484928207641E-16,
-1.));
#7113=DIRECTION('ref_axis',(-1.,-1.60052481607801E-33,1.60923747916479E-15));
#7114=DIRECTION('center_axis',(9.93152043710262E-16,-1.51371712302742E-15,
-1.));
#7115=DIRECTION('ref_axis',(-1.50815602913865E-32,1.,-1.51371712302742E-15));
#7116=DIRECTION('center_axis',(0.,0.,-1.));
#7117=DIRECTION('ref_axis',(-1.,0.,0.));
#7118=DIRECTION('center_axis',(0.,0.,-1.));
#7119=DIRECTION('ref_axis',(-1.,0.,0.));
#7120=DIRECTION('center_axis',(-8.7326569659373E-16,2.3838970357535E-16,
-1.));
#7121=DIRECTION('ref_axis',(-1.,-2.57646307002641E-33,8.7326569659373E-16));
#7122=DIRECTION('center_axis',(6.43084387593756E-16,-6.37075425716023E-16,
-1.));
#7123=DIRECTION('ref_axis',(-1.,-1.009271785482E-32,-6.43084387593756E-16));
#7124=DIRECTION('center_axis',(0.,0.,-1.));
#7125=DIRECTION('ref_axis',(-1.,0.,0.));
#7126=DIRECTION('center_axis',(0.,0.,-1.));
#7127=DIRECTION('ref_axis',(-1.,0.,0.));
#7128=DIRECTION('center_axis',(7.61486879733257E-16,-4.89449036787473E-16,
-1.));
#7129=DIRECTION('ref_axis',(-1.,-8.14289481143214E-33,-7.61486879733257E-16));
#7130=DIRECTION('center_axis',(0.,0.,-1.));
#7131=DIRECTION('ref_axis',(-1.,0.,0.));
#7132=DIRECTION('center_axis',(0.,0.,-1.));
#7133=DIRECTION('ref_axis',(-1.,0.,0.));
#7134=DIRECTION('center_axis',(1.69321748241794E-15,-6.40862752628506E-16,
-1.));
#7135=DIRECTION('ref_axis',(-1.,-4.80921258844117E-33,-1.69321748241794E-15));
#7136=DIRECTION('center_axis',(0.,0.,-1.));
#7137=DIRECTION('ref_axis',(-1.,0.,0.));
#7138=DIRECTION('center_axis',(0.,0.,-1.));
#7139=DIRECTION('ref_axis',(-1.,0.,0.));
#7140=DIRECTION('center_axis',(0.,0.,-1.));
#7141=DIRECTION('ref_axis',(-1.,0.,0.));
#7142=DIRECTION('center_axis',(-8.4660874120897E-16,-3.20431376314254E-16,
-1.));
#7143=DIRECTION('ref_axis',(-1.,-5.07857362029003E-33,8.4660874120897E-16));
#7144=DIRECTION('center_axis',(1.78945947642876E-15,-2.74818654191543E-16,
-1.));
#7145=DIRECTION('ref_axis',(-1.,3.80943324177873E-33,-1.78945947642876E-15));
#7146=DIRECTION('center_axis',(1.16673654887522E-15,-8.66514480280381E-16,
-1.));
#7147=DIRECTION('ref_axis',(-1.,-8.31157122874193E-32,-1.16673654887522E-15));
#7148=DIRECTION('center_axis',(0.,0.,-1.));
#7149=DIRECTION('ref_axis',(-1.,0.,0.));
#7150=DIRECTION('center_axis',(0.,0.,-1.));
#7151=DIRECTION('ref_axis',(-1.,0.,0.));
#7152=DIRECTION('center_axis',(-7.61486879733269E-16,-4.89449036787465E-16,
-1.));
#7153=DIRECTION('ref_axis',(-1.,8.14289481143968E-33,7.61486879733269E-16));
#7154=DIRECTION('center_axis',(1.80749350454039E-15,1.03236338159813E-16,
-1.));
#7155=DIRECTION('ref_axis',(-1.,4.30743575606662E-34,-1.80749350454039E-15));
#7156=DIRECTION('center_axis',(0.,0.,-1.));
#7157=DIRECTION('ref_axis',(-1.,0.,0.));
#7158=DIRECTION('center_axis',(0.,0.,-1.));
#7159=DIRECTION('ref_axis',(-1.,0.,0.));
#7160=DIRECTION('center_axis',(0.,0.,-1.));
#7161=DIRECTION('ref_axis',(-1.,0.,0.));
#7162=DIRECTION('center_axis',(-6.43084387593765E-16,-6.37075425716018E-16,
-1.));
#7163=DIRECTION('ref_axis',(-1.,1.00927178548269E-32,6.43084387593765E-16));
#7164=DIRECTION('center_axis',(1.74653139318747E-15,4.76779407150673E-16,
-1.));
#7165=DIRECTION('ref_axis',(-1.,-8.38515567292817E-33,-1.74653139318747E-15));
#7166=DIRECTION('center_axis',(0.,0.,-1.));
#7167=DIRECTION('ref_axis',(-1.,0.,0.));
#7168=DIRECTION('center_axis',(0.,0.,-1.));
#7169=DIRECTION('ref_axis',(-1.,0.,0.));
#7170=DIRECTION('center_axis',(1.3675338218833E-16,1.44686558860067E-15,
-1.));
#7171=DIRECTION('ref_axis',(2.17929987622515E-32,1.,1.44686558860067E-15));
#7172=DIRECTION('center_axis',(-9.93152043710302E-16,-1.51371712302744E-15,
-1.));
#7173=DIRECTION('ref_axis',(1.50815602913434E-32,1.,-1.51371712302744E-15));
#7174=DIRECTION('center_axis',(1.60923747916481E-15,8.29484928207625E-16,
-1.));
#7175=DIRECTION('ref_axis',(-1.,1.60052481611945E-33,-1.60923747916481E-15));
#7176=DIRECTION('center_axis',(1.45323412840514E-15,-1.52344036793355E-17,
-1.));
#7177=DIRECTION('ref_axis',(-1.,2.33073141122416E-33,-1.45323412840514E-15));
#7178=DIRECTION('center_axis',(0.,0.,-1.));
#7179=DIRECTION('ref_axis',(-1.,0.,0.));
#7180=DIRECTION('center_axis',(0.,0.,-1.));
#7181=DIRECTION('ref_axis',(-1.,0.,0.));
#7182=DIRECTION('center_axis',(-6.56729802250671E-16,-1.68712669272587E-15,
-1.));
#7183=DIRECTION('ref_axis',(-9.28280238059528E-34,1.,-1.68712669272587E-15));
#7184=DIRECTION('center_axis',(1.4016121653245E-15,1.14593797759163E-15,
-1.));
#7185=DIRECTION('ref_axis',(-1.,-1.1095670558325E-32,-1.4016121653245E-15));
#7186=DIRECTION('center_axis',(0.,0.,-1.));
#7187=DIRECTION('ref_axis',(-1.,0.,0.));
#7188=DIRECTION('center_axis',(0.,0.,-1.));
#7189=DIRECTION('ref_axis',(-1.,0.,0.));
#7190=DIRECTION('center_axis',(0.,0.,-1.));
#7191=DIRECTION('ref_axis',(-1.,0.,0.));
#7192=DIRECTION('center_axis',(0.,0.,-1.));
#7193=DIRECTION('ref_axis',(-1.,0.,0.));
#7194=DIRECTION('center_axis',(5.66364837089046E-16,7.06154019267162E-16,
-1.));
#7195=DIRECTION('ref_axis',(-2.86938317198595E-34,1.,7.06154019267162E-16));
#7196=DIRECTION('center_axis',(0.,0.,-1.));
#7197=DIRECTION('ref_axis',(-1.,0.,0.));
#7198=DIRECTION('center_axis',(0.,0.,-1.));
#7199=DIRECTION('ref_axis',(-1.,0.,0.));
#7200=DIRECTION('center_axis',(0.,0.,-1.));
#7201=DIRECTION('ref_axis',(-1.,0.,0.));
#7202=DIRECTION('center_axis',(4.31318598491376E-17,-9.04191500891285E-16,
-1.));
#7203=DIRECTION('ref_axis',(1.09164579340007E-34,1.,-9.04191500891285E-16));
#7204=DIRECTION('center_axis',(4.07170730415051E-16,8.0847673059362E-16,
-1.));
#7205=DIRECTION('ref_axis',(6.01739504655179E-33,1.,8.0847673059362E-16));
#7206=DIRECTION('center_axis',(0.,0.,-1.));
#7207=DIRECTION('ref_axis',(-1.,0.,0.));
#7208=DIRECTION('center_axis',(0.,0.,-1.));
#7209=DIRECTION('ref_axis',(-1.,0.,0.));
#7210=DIRECTION('center_axis',(0.,0.,-1.));
#7211=DIRECTION('ref_axis',(-1.,0.,0.));
#7212=DIRECTION('center_axis',(2.30181308999977E-16,-8.75465129291365E-16,
-1.));
#7213=DIRECTION('ref_axis',(2.99401685849273E-33,1.,-8.75465129291365E-16));
#7214=DIRECTION('center_axis',(2.30181308999981E-16,8.75465129291358E-16,
-1.));
#7215=DIRECTION('ref_axis',(-2.99401685849028E-33,1.,8.75465129291358E-16));
#7216=DIRECTION('center_axis',(9.83724801784613E-16,1.06976961695994E-15,
-1.));
#7217=DIRECTION('ref_axis',(1.03029779618232E-33,1.,1.06976961695994E-15));
#7218=DIRECTION('center_axis',(0.,0.,-1.));
#7219=DIRECTION('ref_axis',(-1.,0.,0.));
#7220=DIRECTION('center_axis',(1.18464566449553E-15,-8.41864697328891E-16,
-1.));
#7221=DIRECTION('ref_axis',(-1.,-9.58283674537864E-32,-1.18464566449553E-15));
#7222=DIRECTION('center_axis',(4.07170730415049E-16,-8.08476730593625E-16,
-1.));
#7223=DIRECTION('ref_axis',(-6.01739504655004E-33,1.,-8.08476730593625E-16));
#7224=DIRECTION('center_axis',(8.62637196982854E-17,1.80838300178258E-15,
-1.));
#7225=DIRECTION('ref_axis',(-4.36658317360796E-34,1.,1.80838300178258E-15));
#7226=DIRECTION('center_axis',(0.,0.,-1.));
#7227=DIRECTION('ref_axis',(-1.,0.,0.));
#7228=DIRECTION('center_axis',(0.,0.,-1.));
#7229=DIRECTION('ref_axis',(-1.,0.,0.));
#7230=DIRECTION('center_axis',(0.,0.,-1.));
#7231=DIRECTION('ref_axis',(-1.,0.,0.));
#7232=DIRECTION('center_axis',(0.,0.,-1.));
#7233=DIRECTION('ref_axis',(-1.,0.,0.));
#7234=DIRECTION('center_axis',(-2.91605317093461E-16,1.78680073022012E-15,
-1.));
#7235=DIRECTION('ref_axis',(-4.81742820615809E-33,1.,1.78680073022012E-15));
#7236=DIRECTION('center_axis',(4.63562821373925E-16,1.3774000978861E-15,
-1.));
#7237=DIRECTION('ref_axis',(1.06074921525595E-31,1.,1.3774000978861E-15));
#7238=DIRECTION('center_axis',(0.,0.,-1.));
#7239=DIRECTION('ref_axis',(-1.,0.,0.));
#7240=DIRECTION('center_axis',(0.,0.,-1.));
#7241=DIRECTION('ref_axis',(-1.,0.,0.));
#7242=DIRECTION('center_axis',(7.00806082662239E-16,-5.72968988795806E-16,
-1.));
#7243=DIRECTION('ref_axis',(-1.,2.77391763959504E-33,-7.00806082662239E-16));
#7244=DIRECTION('center_axis',(0.,0.,-1.));
#7245=DIRECTION('ref_axis',(-1.,0.,0.));
#7246=DIRECTION('center_axis',(0.,0.,-1.));
#7247=DIRECTION('ref_axis',(-1.,0.,0.));
#7248=DIRECTION('center_axis',(0.,0.,-1.));
#7249=DIRECTION('ref_axis',(-1.,0.,0.));
#7250=DIRECTION('center_axis',(0.,0.,-1.));
#7251=DIRECTION('ref_axis',(-1.,0.,0.));
#7252=DIRECTION('',(1.13134139737618E-16,-1.,0.));
#7253=DIRECTION('',(-1.,0.,0.));
#7254=DIRECTION('',(1.13134139737618E-16,1.,0.));
#7255=DIRECTION('center_axis',(0.,0.,-1.));
#7256=DIRECTION('ref_axis',(-1.,0.,0.));
#7257=DIRECTION('',(0.,0.,-1.));
#7258=DIRECTION('center_axis',(0.,0.,1.));
#7259=DIRECTION('ref_axis',(1.,0.,0.));
#7260=DIRECTION('',(0.,0.,1.));
#7261=DIRECTION('center_axis',(0.,0.,1.));
#7262=DIRECTION('ref_axis',(1.,0.,0.));
#7263=DIRECTION('',(0.,0.,-1.));
#7264=DIRECTION('center_axis',(0.,0.,1.));
#7265=DIRECTION('ref_axis',(1.,0.,0.));
#7266=DIRECTION('',(0.,0.,-1.));
#7267=DIRECTION('',(0.,0.,1.));
#7268=DIRECTION('center_axis',(0.,0.,-1.));
#7269=DIRECTION('ref_axis',(-1.,0.,0.));
#7270=DIRECTION('center_axis',(0.,0.,-1.));
#7271=DIRECTION('ref_axis',(-1.,0.,0.));
#7272=DIRECTION('center_axis',(0.,0.,1.));
#7273=DIRECTION('ref_axis',(-0.988411742041742,-0.151796667269113,0.));
#7274=DIRECTION('',(0.,0.,-1.));
#7275=DIRECTION('center_axis',(0.,0.,1.));
#7276=DIRECTION('ref_axis',(1.,0.,0.));
#7277=DIRECTION('',(0.,0.,1.));
#7278=DIRECTION('center_axis',(0.,0.,-1.));
#7279=DIRECTION('ref_axis',(-1.,0.,0.));
#7280=DIRECTION('',(0.,0.,-1.));
#7281=DIRECTION('center_axis',(0.,0.,1.));
#7282=DIRECTION('ref_axis',(1.,0.,0.));
#7283=DIRECTION('',(0.,0.,1.));
#7284=DIRECTION('center_axis',(0.,0.,-1.));
#7285=DIRECTION('ref_axis',(0.802811069346193,0.596233500346318,0.));
#7286=DIRECTION('center_axis',(0.,0.,1.));
#7287=DIRECTION('ref_axis',(1.,0.,0.));
#7288=DIRECTION('center_axis',(0.,0.,1.));
#7289=DIRECTION('ref_axis',(1.,0.,0.));
#7290=DIRECTION('',(0.,0.,1.));
#7291=DIRECTION('center_axis',(0.,0.,-1.));
#7292=DIRECTION('ref_axis',(-1.,0.,0.));
#7293=DIRECTION('',(0.,0.,-1.));
#7294=DIRECTION('center_axis',(0.,0.,1.));
#7295=DIRECTION('ref_axis',(1.,0.,0.));
#7296=DIRECTION('center_axis',(0.,0.,1.));
#7297=DIRECTION('ref_axis',(1.,0.,0.));
#7298=DIRECTION('center_axis',(0.,0.,1.));
#7299=DIRECTION('ref_axis',(1.,0.,0.));
#7300=DIRECTION('',(0.,0.,1.));
#7301=DIRECTION('center_axis',(0.,0.,-1.));
#7302=DIRECTION('ref_axis',(-1.,0.,0.));
#7303=DIRECTION('',(0.,0.,-1.));
#7304=DIRECTION('center_axis',(0.,0.,1.));
#7305=DIRECTION('ref_axis',(1.,0.,0.));
#7306=DIRECTION('center_axis',(0.,0.,1.));
#7307=DIRECTION('ref_axis',(1.,0.,0.));
#7308=DIRECTION('center_axis',(0.,0.,1.));
#7309=DIRECTION('ref_axis',(1.,0.,0.));
#7310=DIRECTION('',(0.,0.,1.));
#7311=DIRECTION('center_axis',(0.,0.,-1.));
#7312=DIRECTION('ref_axis',(-1.,0.,0.));
#7313=DIRECTION('',(0.,0.,-1.));
#7314=DIRECTION('center_axis',(0.,0.,1.));
#7315=DIRECTION('ref_axis',(1.,0.,0.));
#7316=DIRECTION('center_axis',(0.,0.,1.));
#7317=DIRECTION('ref_axis',(1.,0.,0.));
#7318=DIRECTION('center_axis',(0.,0.,1.));
#7319=DIRECTION('ref_axis',(1.,0.,0.));
#7320=DIRECTION('',(0.,0.,1.));
#7321=DIRECTION('center_axis',(0.,0.,-1.));
#7322=DIRECTION('ref_axis',(-1.,0.,0.));
#7323=DIRECTION('',(0.,0.,-1.));
#7324=DIRECTION('center_axis',(0.,0.,1.));
#7325=DIRECTION('ref_axis',(1.,0.,0.));
#7326=DIRECTION('center_axis',(0.,0.,1.));
#7327=DIRECTION('ref_axis',(1.,0.,0.));
#7328=DIRECTION('center_axis',(0.,0.,1.));
#7329=DIRECTION('ref_axis',(1.,0.,0.));
#7330=DIRECTION('',(0.,0.,1.));
#7331=DIRECTION('center_axis',(0.,0.,-1.));
#7332=DIRECTION('ref_axis',(-1.,0.,0.));
#7333=DIRECTION('',(0.,0.,-1.));
#7334=DIRECTION('center_axis',(0.,0.,1.));
#7335=DIRECTION('ref_axis',(1.,0.,0.));
#7336=DIRECTION('center_axis',(0.,0.,1.));
#7337=DIRECTION('ref_axis',(1.,0.,0.));
#7338=DIRECTION('',(0.,0.,-1.));
#7339=DIRECTION('center_axis',(0.,0.,1.));
#7340=DIRECTION('ref_axis',(1.,0.,0.));
#7341=DIRECTION('center_axis',(0.,0.,1.));
#7342=DIRECTION('ref_axis',(1.,0.,0.));
#7343=DIRECTION('',(0.,0.,1.));
#7344=DIRECTION('center_axis',(0.,0.,-1.));
#7345=DIRECTION('ref_axis',(-1.,0.,0.));
#7346=DIRECTION('center_axis',(0.,0.,1.));
#7347=DIRECTION('ref_axis',(1.,0.,0.));
#7348=DIRECTION('',(0.,0.,-1.));
#7349=DIRECTION('center_axis',(0.,0.,1.));
#7350=DIRECTION('ref_axis',(1.,0.,0.));
#7351=DIRECTION('center_axis',(0.,0.,1.));
#7352=DIRECTION('ref_axis',(1.,0.,0.));
#7353=DIRECTION('',(0.,0.,1.));
#7354=DIRECTION('center_axis',(0.,0.,-1.));
#7355=DIRECTION('ref_axis',(-1.,0.,0.));
#7356=DIRECTION('center_axis',(0.,0.,1.));
#7357=DIRECTION('ref_axis',(1.,0.,0.));
#7358=DIRECTION('',(0.,0.,-1.));
#7359=DIRECTION('center_axis',(0.,0.,1.));
#7360=DIRECTION('ref_axis',(1.,0.,0.));
#7361=DIRECTION('center_axis',(0.,0.,1.));
#7362=DIRECTION('ref_axis',(1.,0.,0.));
#7363=DIRECTION('',(0.,0.,1.));
#7364=DIRECTION('center_axis',(0.,0.,-1.));
#7365=DIRECTION('ref_axis',(-1.,0.,0.));
#7366=DIRECTION('center_axis',(0.,0.,1.));
#7367=DIRECTION('ref_axis',(1.,0.,0.));
#7368=DIRECTION('',(0.,0.,-1.));
#7369=DIRECTION('center_axis',(0.,0.,1.));
#7370=DIRECTION('ref_axis',(1.,0.,0.));
#7371=DIRECTION('center_axis',(0.,0.,1.));
#7372=DIRECTION('ref_axis',(1.,0.,0.));
#7373=DIRECTION('',(0.,0.,1.));
#7374=DIRECTION('center_axis',(0.,0.,-1.));
#7375=DIRECTION('ref_axis',(-1.,0.,0.));
#7376=DIRECTION('center_axis',(0.,0.,1.));
#7377=DIRECTION('ref_axis',(1.,0.,0.));
#7378=DIRECTION('',(0.,0.,-1.));
#7379=DIRECTION('center_axis',(0.,0.,1.));
#7380=DIRECTION('ref_axis',(1.,0.,0.));
#7381=DIRECTION('center_axis',(0.,0.,1.));
#7382=DIRECTION('ref_axis',(1.,0.,0.));
#7383=DIRECTION('',(0.,0.,1.));
#7384=DIRECTION('center_axis',(0.,0.,-1.));
#7385=DIRECTION('ref_axis',(-1.,0.,0.));
#7386=DIRECTION('center_axis',(0.,0.,1.));
#7387=DIRECTION('ref_axis',(1.,0.,0.));
#7388=DIRECTION('',(0.,0.,-1.));
#7389=DIRECTION('center_axis',(0.,0.,1.));
#7390=DIRECTION('ref_axis',(1.,0.,0.));
#7391=DIRECTION('',(0.,0.,1.));
#7392=DIRECTION('center_axis',(0.,0.,-1.));
#7393=DIRECTION('ref_axis',(-1.,0.,0.));
#7394=DIRECTION('center_axis',(0.,0.,1.));
#7395=DIRECTION('ref_axis',(1.,0.,0.));
#7396=DIRECTION('',(0.,0.,-1.));
#7397=DIRECTION('center_axis',(0.,0.,1.));
#7398=DIRECTION('ref_axis',(1.,0.,0.));
#7399=DIRECTION('',(0.,0.,1.));
#7400=DIRECTION('center_axis',(0.,0.,-1.));
#7401=DIRECTION('ref_axis',(-1.,0.,0.));
#7402=DIRECTION('center_axis',(0.,0.,1.));
#7403=DIRECTION('ref_axis',(1.,0.,0.));
#7404=DIRECTION('',(0.,0.,1.));
#7405=DIRECTION('center_axis',(0.,0.,-1.));
#7406=DIRECTION('ref_axis',(-1.,0.,0.));
#7407=DIRECTION('',(0.,0.,-1.));
#7408=DIRECTION('center_axis',(0.,0.,1.));
#7409=DIRECTION('ref_axis',(1.,0.,0.));
#7410=DIRECTION('center_axis',(0.,0.,1.));
#7411=DIRECTION('ref_axis',(1.,0.,0.));
#7412=DIRECTION('',(0.,0.,1.));
#7413=DIRECTION('center_axis',(0.,0.,-1.));
#7414=DIRECTION('ref_axis',(-1.,0.,0.));
#7415=DIRECTION('',(0.,0.,-1.));
#7416=DIRECTION('center_axis',(0.,0.,1.));
#7417=DIRECTION('ref_axis',(1.,0.,0.));
#7418=DIRECTION('center_axis',(0.,0.,1.));
#7419=DIRECTION('ref_axis',(1.,0.,0.));
#7420=DIRECTION('',(0.,0.,-1.));
#7421=DIRECTION('center_axis',(0.,0.,1.));
#7422=DIRECTION('ref_axis',(1.,0.,0.));
#7423=DIRECTION('',(0.,0.,1.));
#7424=DIRECTION('center_axis',(0.,0.,-1.));
#7425=DIRECTION('ref_axis',(-1.,0.,0.));
#7426=DIRECTION('',(0.,0.,-1.));
#7427=DIRECTION('center_axis',(0.,0.,1.));
#7428=DIRECTION('ref_axis',(1.,0.,0.));
#7429=DIRECTION('',(0.,0.,1.));
#7430=DIRECTION('center_axis',(0.,0.,-1.));
#7431=DIRECTION('ref_axis',(-1.,0.,0.));
#7432=DIRECTION('center_axis',(0.,0.,1.));
#7433=DIRECTION('ref_axis',(1.,0.,0.));
#7434=DIRECTION('',(0.,0.,-1.));
#7435=DIRECTION('center_axis',(0.,0.,1.));
#7436=DIRECTION('ref_axis',(-0.98841174204174,0.151796667269121,0.));
#7437=DIRECTION('',(0.,0.,1.));
#7438=DIRECTION('center_axis',(0.,0.,-1.));
#7439=DIRECTION('ref_axis',(0.802811069346192,-0.596233500346319,0.));
#7440=DIRECTION('',(0.,0.,-1.));
#7441=DIRECTION('center_axis',(0.,0.,1.));
#7442=DIRECTION('ref_axis',(1.,0.,0.));
#7443=DIRECTION('',(0.,0.,1.));
#7444=DIRECTION('center_axis',(0.,0.,-1.));
#7445=DIRECTION('ref_axis',(-1.,0.,0.));
#7446=DIRECTION('center_axis',(0.,0.,1.));
#7447=DIRECTION('ref_axis',(1.,0.,0.));
#7448=DIRECTION('',(0.,0.,-1.));
#7449=DIRECTION('center_axis',(0.,0.,1.));
#7450=DIRECTION('ref_axis',(1.,0.,0.));
#7451=DIRECTION('',(0.,0.,1.));
#7452=DIRECTION('center_axis',(0.,0.,-1.));
#7453=DIRECTION('ref_axis',(0.999945056799679,-0.0104825274569905,0.));
#7454=DIRECTION('',(0.,0.,-1.));
#7455=DIRECTION('center_axis',(0.,0.,1.));
#7456=DIRECTION('ref_axis',(1.,0.,0.));
#7457=DIRECTION('',(0.,0.,1.));
#7458=DIRECTION('center_axis',(0.,0.,-1.));
#7459=DIRECTION('ref_axis',(-1.,0.,0.));
#7460=DIRECTION('center_axis',(0.,0.,1.));
#7461=DIRECTION('ref_axis',(1.,0.,0.));
#7462=DIRECTION('',(0.,0.,-1.));
#7463=DIRECTION('center_axis',(0.,0.,1.));
#7464=DIRECTION('ref_axis',(1.,0.,0.));
#7465=DIRECTION('',(0.,0.,1.));
#7466=DIRECTION('center_axis',(0.,0.,-1.));
#7467=DIRECTION('ref_axis',(0.980273298181862,0.1976468084024,0.));
#7468=DIRECTION('',(0.,0.,-1.));
#7469=DIRECTION('center_axis',(0.,0.,1.));
#7470=DIRECTION('ref_axis',(1.,0.,0.));
#7471=DIRECTION('',(0.,0.,1.));
#7472=DIRECTION('center_axis',(0.,0.,-1.));
#7473=DIRECTION('ref_axis',(-1.,0.,0.));
#7474=DIRECTION('center_axis',(0.,0.,1.));
#7475=DIRECTION('ref_axis',(1.,0.,0.));
#7476=DIRECTION('',(0.,0.,-1.));
#7477=DIRECTION('center_axis',(0.,0.,1.));
#7478=DIRECTION('ref_axis',(1.,0.,0.));
#7479=DIRECTION('',(0.,0.,1.));
#7480=DIRECTION('center_axis',(0.,0.,-1.));
#7481=DIRECTION('ref_axis',(0.975914418166608,-0.218153726565768,0.));
#7482=DIRECTION('',(0.,0.,-1.));
#7483=DIRECTION('center_axis',(0.,0.,1.));
#7484=DIRECTION('ref_axis',(1.,0.,0.));
#7485=DIRECTION('',(0.,0.,1.));
#7486=DIRECTION('center_axis',(0.,0.,-1.));
#7487=DIRECTION('ref_axis',(-1.,0.,0.));
#7488=DIRECTION('center_axis',(0.,0.,1.));
#7489=DIRECTION('ref_axis',(1.,0.,0.));
#7490=DIRECTION('',(0.,0.,-1.));
#7491=DIRECTION('center_axis',(0.,0.,1.));
#7492=DIRECTION('ref_axis',(-0.998372875767673,-0.0570228106233482,0.));
#7493=DIRECTION('',(0.,0.,1.));
#7494=DIRECTION('center_axis',(0.,0.,-1.));
#7495=DIRECTION('ref_axis',(0.909231636502713,-0.416290561005889,0.));
#7496=DIRECTION('',(0.,0.,-1.));
#7497=DIRECTION('center_axis',(0.,0.,1.));
#7498=DIRECTION('ref_axis',(1.,0.,0.));
#7499=DIRECTION('',(0.,0.,1.));
#7500=DIRECTION('center_axis',(0.,0.,-1.));
#7501=DIRECTION('ref_axis',(-1.,0.,0.));
#7502=DIRECTION('center_axis',(0.,0.,1.));
#7503=DIRECTION('ref_axis',(1.,0.,0.));
#7504=DIRECTION('',(0.,0.,-1.));
#7505=DIRECTION('center_axis',(0.,0.,1.));
#7506=DIRECTION('ref_axis',(1.,0.,0.));
#7507=DIRECTION('',(0.,0.,1.));
#7508=DIRECTION('center_axis',(0.,0.,-1.));
#7509=DIRECTION('ref_axis',(0.917758892560327,0.397138030319992,0.));
#7510=DIRECTION('',(0.,0.,-1.));
#7511=DIRECTION('center_axis',(0.,0.,1.));
#7512=DIRECTION('ref_axis',(1.,0.,0.));
#7513=DIRECTION('',(0.,0.,1.));
#7514=DIRECTION('center_axis',(0.,0.,-1.));
#7515=DIRECTION('ref_axis',(-1.,0.,0.));
#7516=DIRECTION('center_axis',(0.,0.,1.));
#7517=DIRECTION('ref_axis',(1.,0.,0.));
#7518=DIRECTION('',(0.,0.,-1.));
#7519=DIRECTION('center_axis',(0.,0.,1.));
#7520=DIRECTION('ref_axis',(1.,0.,0.));
#7521=DIRECTION('',(0.,0.,1.));
#7522=DIRECTION('center_axis',(0.,0.,-1.));
#7523=DIRECTION('ref_axis',(0.815134019438133,0.579272414632902,0.));
#7524=DIRECTION('',(0.,0.,-1.));
#7525=DIRECTION('center_axis',(0.,0.,1.));
#7526=DIRECTION('ref_axis',(1.,0.,0.));
#7527=DIRECTION('',(0.,0.,1.));
#7528=DIRECTION('center_axis',(0.,0.,-1.));
#7529=DIRECTION('ref_axis',(-1.,0.,0.));
#7530=DIRECTION('center_axis',(0.,0.,1.));
#7531=DIRECTION('ref_axis',(1.,0.,0.));
#7532=DIRECTION('',(0.,0.,-1.));
#7533=DIRECTION('center_axis',(0.,0.,1.));
#7534=DIRECTION('ref_axis',(1.,0.,0.));
#7535=DIRECTION('',(0.,0.,1.));
#7536=DIRECTION('center_axis',(0.,0.,-1.));
#7537=DIRECTION('ref_axis',(-1.,0.,0.));
#7538=DIRECTION('',(0.,0.,-1.));
#7539=DIRECTION('center_axis',(0.,0.,1.));
#7540=DIRECTION('ref_axis',(1.,0.,0.));
#7541=DIRECTION('',(0.,0.,1.));
#7542=DIRECTION('center_axis',(0.,0.,-1.));
#7543=DIRECTION('ref_axis',(0.815134019438124,-0.579272414632915,0.));
#7544=DIRECTION('center_axis',(0.,0.,1.));
#7545=DIRECTION('ref_axis',(1.,0.,0.));
#7546=DIRECTION('',(0.,0.,-1.));
#7547=DIRECTION('center_axis',(0.,0.,1.));
#7548=DIRECTION('ref_axis',(1.,0.,0.));
#7549=DIRECTION('',(0.,0.,1.));
#7550=DIRECTION('center_axis',(0.,0.,-1.));
#7551=DIRECTION('ref_axis',(-1.,0.,0.));
#7552=DIRECTION('',(0.,0.,-1.));
#7553=DIRECTION('center_axis',(0.,0.,1.));
#7554=DIRECTION('ref_axis',(1.,0.,0.));
#7555=DIRECTION('',(0.,0.,1.));
#7556=DIRECTION('center_axis',(0.,0.,-1.));
#7557=DIRECTION('ref_axis',(0.917758892560322,-0.397138030320002,0.));
#7558=DIRECTION('center_axis',(0.,0.,1.));
#7559=DIRECTION('ref_axis',(-0.998372875767673,0.0570228106233547,0.));
#7560=DIRECTION('',(0.,0.,-1.));
#7561=DIRECTION('center_axis',(0.,0.,1.));
#7562=DIRECTION('ref_axis',(1.,0.,0.));
#7563=DIRECTION('',(0.,0.,1.));
#7564=DIRECTION('center_axis',(0.,0.,-1.));
#7565=DIRECTION('ref_axis',(-1.,0.,0.));
#7566=DIRECTION('',(0.,0.,-1.));
#7567=DIRECTION('center_axis',(0.,0.,1.));
#7568=DIRECTION('ref_axis',(1.,0.,0.));
#7569=DIRECTION('',(0.,0.,1.));
#7570=DIRECTION('center_axis',(0.,0.,-1.));
#7571=DIRECTION('ref_axis',(0.909231636502717,0.416290561005881,0.));
#7572=DIRECTION('center_axis',(0.,0.,1.));
#7573=DIRECTION('ref_axis',(1.,0.,0.));
#7574=DIRECTION('',(0.,0.,-1.));
#7575=DIRECTION('center_axis',(0.,0.,1.));
#7576=DIRECTION('ref_axis',(1.,0.,0.));
#7577=DIRECTION('',(0.,0.,1.));
#7578=DIRECTION('center_axis',(0.,0.,-1.));
#7579=DIRECTION('ref_axis',(-1.,0.,0.));
#7580=DIRECTION('',(0.,0.,-1.));
#7581=DIRECTION('center_axis',(0.,0.,1.));
#7582=DIRECTION('ref_axis',(1.,0.,0.));
#7583=DIRECTION('',(0.,0.,1.));
#7584=DIRECTION('center_axis',(0.,0.,-1.));
#7585=DIRECTION('ref_axis',(0.975914418166611,0.218153726565752,0.));
#7586=DIRECTION('center_axis',(0.,0.,1.));
#7587=DIRECTION('ref_axis',(1.,0.,0.));
#7588=DIRECTION('',(0.,0.,-1.));
#7589=DIRECTION('center_axis',(0.,0.,1.));
#7590=DIRECTION('ref_axis',(1.,0.,0.));
#7591=DIRECTION('',(0.,0.,1.));
#7592=DIRECTION('center_axis',(0.,0.,-1.));
#7593=DIRECTION('ref_axis',(-1.,0.,0.));
#7594=DIRECTION('',(0.,0.,-1.));
#7595=DIRECTION('center_axis',(0.,0.,1.));
#7596=DIRECTION('ref_axis',(1.,0.,0.));
#7597=DIRECTION('',(0.,0.,1.));
#7598=DIRECTION('center_axis',(0.,0.,-1.));
#7599=DIRECTION('ref_axis',(0.98027329818186,-0.19764680840241,0.));
#7600=DIRECTION('center_axis',(0.,0.,1.));
#7601=DIRECTION('ref_axis',(1.,0.,0.));
#7602=DIRECTION('',(0.,0.,-1.));
#7603=DIRECTION('center_axis',(0.,0.,1.));
#7604=DIRECTION('ref_axis',(1.,0.,0.));
#7605=DIRECTION('',(0.,0.,1.));
#7606=DIRECTION('center_axis',(0.,0.,-1.));
#7607=DIRECTION('ref_axis',(-1.,0.,0.));
#7608=DIRECTION('',(0.,0.,-1.));
#7609=DIRECTION('center_axis',(0.,0.,1.));
#7610=DIRECTION('ref_axis',(1.,0.,0.));
#7611=DIRECTION('',(0.,0.,1.));
#7612=DIRECTION('center_axis',(0.,0.,-1.));
#7613=DIRECTION('ref_axis',(0.999945056799679,0.010482527456989,0.));
#7614=DIRECTION('center_axis',(0.,1.,0.));
#7615=DIRECTION('ref_axis',(0.,0.,1.));
#7616=DIRECTION('',(0.,0.,1.));
#7617=DIRECTION('',(0.,0.,1.));
#7618=DIRECTION('center_axis',(-1.,-1.13134139737618E-16,0.));
#7619=DIRECTION('ref_axis',(1.13134139737618E-16,-1.,0.));
#7620=DIRECTION('center_axis',(1.,-1.13134139737618E-16,0.));
#7621=DIRECTION('ref_axis',(1.13134139737618E-16,1.,0.));
#8113=CARTESIAN_POINT('',(0.,0.,0.));
#8114=CARTESIAN_POINT('Origin',(3.51281503885303E-14,-0.121376657232176,
-0.999999999999996));
#8115=CARTESIAN_POINT('',(-1.49999999999993,4.12126402988712,-0.999999999999996));
#8116=CARTESIAN_POINT('',(1.49999999999993,4.12126402988715,-0.999999999999996));
#8117=CARTESIAN_POINT('Origin',(3.43987251108903E-14,-0.121376657232172,
-0.999999999999996));
#8118=CARTESIAN_POINT('',(-1.49999999999993,4.12126402988712,1.));
#8119=CARTESIAN_POINT('',(-1.49999999999993,4.12126402988712,-0.999999999999996));
#8120=CARTESIAN_POINT('',(1.49999999999993,4.12126402988715,1.));
#8121=CARTESIAN_POINT('Origin',(3.43987251108903E-14,-0.121376657232172,
1.));
#8122=CARTESIAN_POINT('',(1.49999999999993,4.12126402988715,-0.999999999999996));
#8123=CARTESIAN_POINT('Origin',(3.59548358424103,18.5022254123314,-0.999999999999996));
#8124=CARTESIAN_POINT('',(3.51871169276258,18.1045684286397,1.));
#8125=CARTESIAN_POINT('',(3.19260839230423,18.5436570394041,1.));
#8126=CARTESIAN_POINT('Origin',(3.59548358424103,18.5022254123314,1.));
#8127=CARTESIAN_POINT('',(3.51871169276258,18.1045684286397,-0.999999999999996));
#8128=CARTESIAN_POINT('',(3.51871169276258,18.1045684286397,-0.999999999999996));
#8129=CARTESIAN_POINT('',(3.19260839230423,18.5436570394041,-0.999999999999996));
#8130=CARTESIAN_POINT('Origin',(3.59548358424104,18.5022254123314,-0.999999999999996));
#8131=CARTESIAN_POINT('',(3.19260839230423,18.5436570394041,-0.999999999999996));
#8132=CARTESIAN_POINT('Origin',(-2.30964438172635,19.1095079271131,-0.999999999999996));
#8133=CARTESIAN_POINT('',(2.76924223657526,21.3003715775681,-0.999999999999996));
#8134=CARTESIAN_POINT('Origin',(-2.30964438172635,19.1095079271131,-1.00000000000001));
#8135=CARTESIAN_POINT('',(2.76924223657527,21.3003715775681,1.));
#8136=CARTESIAN_POINT('',(2.76924223657526,21.3003715775681,4.082419099807E-15));
#8137=CARTESIAN_POINT('Origin',(-2.30964438172635,19.1095079271131,1.00000000000001));
#8138=CARTESIAN_POINT('Origin',(7.38897823680324,17.3477119528255,-0.999999999999996));
#8139=CARTESIAN_POINT('',(7.23120645950496,16.974706502077,1.));
#8140=CARTESIAN_POINT('',(7.0035209540531,17.4720006617853,1.));
#8141=CARTESIAN_POINT('Origin',(7.38897823680324,17.3477119528255,1.));
#8142=CARTESIAN_POINT('',(7.23120645950496,16.974706502077,-0.999999999999996));
#8143=CARTESIAN_POINT('',(7.23120645950496,16.974706502077,-0.999999999999996));
#8144=CARTESIAN_POINT('',(7.0035209540531,17.4720006617853,-0.999999999999996));
#8145=CARTESIAN_POINT('Origin',(7.38897823680324,17.3477119528255,-0.999999999999996));
#8146=CARTESIAN_POINT('',(7.0035209540531,17.4720006617853,-0.999999999999996));
#8147=CARTESIAN_POINT('Origin',(1.73915261931847,19.1694690275263,-0.999999999999996));
#8148=CARTESIAN_POINT('',(7.16255954532649,20.256497146471,-0.999999999999996));
#8149=CARTESIAN_POINT('Origin',(1.73915261931847,19.1694690275263,-1.));
#8150=CARTESIAN_POINT('',(7.1625595453265,20.256497146471,1.));
#8151=CARTESIAN_POINT('',(7.16255954532649,20.256497146471,4.082419099807E-15));
#8152=CARTESIAN_POINT('Origin',(1.73915261931844,19.1694690275263,1.00000000000001));
#8153=CARTESIAN_POINT('Origin',(3.59548358424065,-18.7449787267958,-0.999999999999996));
#8154=CARTESIAN_POINT('',(3.19260839230386,-18.7864103538685,1.));
#8155=CARTESIAN_POINT('',(3.5187116927622,-18.3473217431041,1.));
#8156=CARTESIAN_POINT('Origin',(3.59548358424064,-18.7449787267958,1.));
#8157=CARTESIAN_POINT('',(3.19260839230386,-18.7864103538685,-0.999999999999996));
#8158=CARTESIAN_POINT('',(3.19260839230386,-18.7864103538685,-0.999999999999996));
#8159=CARTESIAN_POINT('',(3.5187116927622,-18.3473217431041,-0.999999999999996));
#8160=CARTESIAN_POINT('Origin',(3.59548358424064,-18.7449787267958,-0.999999999999996));
#8161=CARTESIAN_POINT('',(3.5187116927622,-18.3473217431041,-0.999999999999996));
#8162=CARTESIAN_POINT('Origin',(-2.30964438172673,-19.3522612415774,-0.999999999999996));
#8163=CARTESIAN_POINT('',(2.76924223657483,-21.5431248920325,-0.999999999999996));
#8164=CARTESIAN_POINT('Origin',(-2.30964438172671,-19.3522612415774,-1.));
#8165=CARTESIAN_POINT('',(2.76924223657484,-21.5431248920325,1.));
#8166=CARTESIAN_POINT('Origin',(-2.30964438172672,-19.3522612415774,1.00000000000001));
#8167=CARTESIAN_POINT('',(2.76924223657483,-21.5431248920325,4.082419099807E-15));
#8168=CARTESIAN_POINT('Origin',(7.38897823680289,-17.59046526729,-0.999999999999996));
#8169=CARTESIAN_POINT('',(7.00352095405275,-17.7147539762498,1.));
#8170=CARTESIAN_POINT('',(7.23120645950461,-17.2174598165415,1.));
#8171=CARTESIAN_POINT('Origin',(7.38897823680288,-17.5904652672901,1.));
#8172=CARTESIAN_POINT('',(7.00352095405275,-17.7147539762498,-0.999999999999996));
#8173=CARTESIAN_POINT('',(7.00352095405275,-17.7147539762498,-0.999999999999996));
#8174=CARTESIAN_POINT('',(7.23120645950461,-17.2174598165415,-0.999999999999996));
#8175=CARTESIAN_POINT('Origin',(7.38897823680288,-17.59046526729,-0.999999999999996));
#8176=CARTESIAN_POINT('',(7.23120645950461,-17.2174598165415,-0.999999999999996));
#8177=CARTESIAN_POINT('Origin',(1.73915261931808,-19.4122223419907,-0.999999999999996));
#8178=CARTESIAN_POINT('',(7.16255954532608,-20.4992504609355,-0.999999999999996));
#8179=CARTESIAN_POINT('Origin',(1.73915261931809,-19.4122223419907,-1.00000000000001));
#8180=CARTESIAN_POINT('',(7.16255954532609,-20.4992504609355,1.));
#8181=CARTESIAN_POINT('Origin',(1.73915261931808,-19.4122223419907,1.00000000000001));
#8182=CARTESIAN_POINT('',(7.16255954532608,-20.4992504609355,4.082419099807E-15));
#8183=CARTESIAN_POINT('Origin',(13.8554859637,-13.0748150023093,-0.999999999999996));
#8184=CARTESIAN_POINT('',(13.5539059861828,-13.3451379890507,1.));
#8185=CARTESIAN_POINT('',(13.5596392883185,-12.7982291301724,1.));
#8186=CARTESIAN_POINT('Origin',(13.8554859637,-13.0748150023093,1.));
#8187=CARTESIAN_POINT('',(13.5539059861828,-13.3451379890507,-0.999999999999996));
#8188=CARTESIAN_POINT('',(13.5539059861828,-13.3451379890507,-0.999999999999996));
#8189=CARTESIAN_POINT('',(13.5596392883185,-12.7982291301724,-0.999999999999996));
#8190=CARTESIAN_POINT('Origin',(13.8554859637,-13.0748150023093,-0.999999999999996));
#8191=CARTESIAN_POINT('',(13.5596392883185,-12.7982291301724,-0.999999999999996));
#8192=CARTESIAN_POINT('Origin',(10.8595390841654,-15.6724688095372,-0.999999999999996));
#8193=CARTESIAN_POINT('',(10.5083460434874,-15.8741825873991,1.));
#8194=CARTESIAN_POINT('',(10.6276628047883,-15.3404170198083,1.));
#8195=CARTESIAN_POINT('Origin',(10.8595390841655,-15.6724688095372,1.));
#8196=CARTESIAN_POINT('',(10.5083460434874,-15.8741825873991,-0.999999999999996));
#8197=CARTESIAN_POINT('',(10.5083460434874,-15.8741825873991,-0.999999999999996));
#8198=CARTESIAN_POINT('',(10.6276628047883,-15.3404170198083,-0.999999999999996));
#8199=CARTESIAN_POINT('Origin',(10.8595390841655,-15.6724688095372,-0.999999999999996));
#8200=CARTESIAN_POINT('',(10.6276628047883,-15.3404170198083,-0.999999999999996));
#8201=CARTESIAN_POINT('Origin',(16.2458816206226,-9.91103378190805,-0.999999999999996));
#8202=CARTESIAN_POINT('',(16.0070951984252,-10.2381515658547,1.));
#8203=CARTESIAN_POINT('',(15.8989944685809,-9.70200195718188,1.));
#8204=CARTESIAN_POINT('Origin',(16.2458816206226,-9.91103378190806,1.));
#8205=CARTESIAN_POINT('',(16.0070951984252,-10.2381515658547,-0.999999999999996));
#8206=CARTESIAN_POINT('',(16.0070951984252,-10.2381515658547,-0.999999999999996));
#8207=CARTESIAN_POINT('',(15.8989944685809,-9.70200195718188,-0.999999999999996));
#8208=CARTESIAN_POINT('Origin',(16.2458816206226,-9.91103378190805,-0.999999999999996));
#8209=CARTESIAN_POINT('',(15.8989944685809,-9.70200195718188,-0.999999999999996));
#8210=CARTESIAN_POINT('Origin',(17.9262542943349,-6.31939756917167,-0.999999999999996));
#8211=CARTESIAN_POINT('',(17.7606975399316,-6.68901353347981,1.));
#8212=CARTESIAN_POINT('',(17.5434872987264,-6.18705548564272,1.));
#8213=CARTESIAN_POINT('Origin',(17.9262542943349,-6.31939756917167,1.));
#8214=CARTESIAN_POINT('',(17.7606975399316,-6.68901353347981,-0.999999999999996));
#8215=CARTESIAN_POINT('',(17.7606975399316,-6.68901353347981,-0.999999999999996));
#8216=CARTESIAN_POINT('',(17.5434872987264,-6.18705548564272,-0.999999999999996));
#8217=CARTESIAN_POINT('Origin',(17.9262542943349,-6.31939756917167,-0.999999999999996));
#8218=CARTESIAN_POINT('',(17.5434872987264,-6.18705548564272,-0.999999999999996));
#8219=CARTESIAN_POINT('Origin',(18.823163635673,-2.45687810117945,-0.999999999999996));
#8220=CARTESIAN_POINT('',(18.7380721736606,-2.85283825459467,1.));
#8221=CARTESIAN_POINT('',(18.4212455509255,-2.4070097429457,1.));
#8222=CARTESIAN_POINT('Origin',(18.823163635673,-2.45687810117946,1.));
#8223=CARTESIAN_POINT('',(18.7380721736606,-2.85283825459467,-0.999999999999996));
#8224=CARTESIAN_POINT('',(18.7380721736606,-2.85283825459467,-0.999999999999996));
#8225=CARTESIAN_POINT('',(18.4212455509255,-2.4070097429457,-0.999999999999996));
#8226=CARTESIAN_POINT('Origin',(18.823163635673,-2.45687810117946,-0.999999999999996));
#8227=CARTESIAN_POINT('',(18.4212455509255,-2.4070097429457,-0.999999999999996));
#8228=CARTESIAN_POINT('Origin',(18.823163635673,2.21412478671471,-0.999999999999996));
#8229=CARTESIAN_POINT('',(18.4212455509256,2.16425642848097,1.));
#8230=CARTESIAN_POINT('',(18.7380721736607,2.61008494012994,1.));
#8231=CARTESIAN_POINT('Origin',(18.823163635673,2.21412478671472,1.));
#8232=CARTESIAN_POINT('',(18.4212455509256,2.16425642848097,-0.999999999999996));
#8233=CARTESIAN_POINT('',(18.4212455509256,2.16425642848097,-0.999999999999996));
#8234=CARTESIAN_POINT('',(18.7380721736607,2.61008494012994,-0.999999999999996));
#8235=CARTESIAN_POINT('Origin',(18.823163635673,2.21412478671472,-0.999999999999996));
#8236=CARTESIAN_POINT('',(18.7380721736607,2.61008494012994,-0.999999999999996));
#8237=CARTESIAN_POINT('Origin',(13.8554859637002,12.8320616878447,-0.999999999999996));
#8238=CARTESIAN_POINT('',(13.5596392883187,12.5554758157078,1.));
#8239=CARTESIAN_POINT('',(13.5539059861831,13.102384674586,1.));
#8240=CARTESIAN_POINT('Origin',(13.8554859637002,12.8320616878447,1.));
#8241=CARTESIAN_POINT('',(13.5596392883187,12.5554758157078,-0.999999999999996));
#8242=CARTESIAN_POINT('',(13.5596392883187,12.5554758157078,-0.999999999999996));
#8243=CARTESIAN_POINT('',(13.5539059861831,13.102384674586,-0.999999999999996));
#8244=CARTESIAN_POINT('Origin',(13.8554859637002,12.8320616878447,-0.999999999999996));
#8245=CARTESIAN_POINT('',(13.5539059861831,13.102384674586,-0.999999999999996));
#8246=CARTESIAN_POINT('Origin',(10.8595390841658,15.4297154950726,-0.999999999999996));
#8247=CARTESIAN_POINT('',(10.6276628047886,15.0976637053437,1.));
#8248=CARTESIAN_POINT('',(10.5083460434877,15.6314292729346,1.));
#8249=CARTESIAN_POINT('Origin',(10.8595390841658,15.4297154950726,1.));
#8250=CARTESIAN_POINT('',(10.6276628047886,15.0976637053437,-0.999999999999996));
#8251=CARTESIAN_POINT('',(10.6276628047886,15.0976637053437,-0.999999999999996));
#8252=CARTESIAN_POINT('',(10.5083460434877,15.6314292729346,-0.999999999999996));
#8253=CARTESIAN_POINT('Origin',(10.8595390841658,15.4297154950726,-0.999999999999996));
#8254=CARTESIAN_POINT('',(10.5083460434877,15.6314292729346,-0.999999999999996));
#8255=CARTESIAN_POINT('Origin',(16.2458816206228,9.66828046744336,-0.999999999999996));
#8256=CARTESIAN_POINT('',(15.8989944685811,9.45924864271719,1.));
#8257=CARTESIAN_POINT('',(16.0070951984254,9.99539825138999,1.));
#8258=CARTESIAN_POINT('Origin',(16.2458816206228,9.66828046744336,1.));
#8259=CARTESIAN_POINT('',(15.8989944685811,9.45924864271719,-0.999999999999996));
#8260=CARTESIAN_POINT('',(15.8989944685811,9.45924864271719,-0.999999999999996));
#8261=CARTESIAN_POINT('',(16.0070951984254,9.99539825138999,-0.999999999999996));
#8262=CARTESIAN_POINT('Origin',(16.2458816206228,9.66828046744336,-0.999999999999995));
#8263=CARTESIAN_POINT('',(16.0070951984254,9.99539825138999,-0.999999999999996));
#8264=CARTESIAN_POINT('Origin',(17.9262542943351,6.07664425470695,-0.999999999999996));
#8265=CARTESIAN_POINT('',(17.5434872987265,5.944302171178,1.));
#8266=CARTESIAN_POINT('',(17.7606975399317,6.4462602190151,1.));
#8267=CARTESIAN_POINT('Origin',(17.9262542943351,6.07664425470695,1.));
#8268=CARTESIAN_POINT('',(17.5434872987265,5.944302171178,-0.999999999999996));
#8269=CARTESIAN_POINT('',(17.5434872987265,5.944302171178,-0.999999999999996));
#8270=CARTESIAN_POINT('',(17.7606975399317,6.4462602190151,-0.999999999999996));
#8271=CARTESIAN_POINT('Origin',(17.9262542943351,6.07664425470695,-0.999999999999996));
#8272=CARTESIAN_POINT('',(17.7606975399317,6.4462602190151,-0.999999999999996));
#8273=CARTESIAN_POINT('Origin',(3.64291929955129E-14,-0.121376657232174,
1.));
#8274=CARTESIAN_POINT('',(-21.5938622919806,0.393512957130182,1.));
#8275=CARTESIAN_POINT('',(-21.5938622919806,-0.636266271594385,1.));
#8276=CARTESIAN_POINT('Origin',(6.93889390390723E-12,-0.1213766572321,1.00000000000115));
#8277=CARTESIAN_POINT('',(-21.5938622919806,0.393512957130176,-0.999999999999996));
#8278=CARTESIAN_POINT('',(-21.5938622919806,0.393512957130177,4.082419099807E-15));
#8279=CARTESIAN_POINT('',(-21.5938622919806,-0.636266271594384,-0.999999999999996));
#8280=CARTESIAN_POINT('Origin',(-2.61943244872498E-12,-0.1213766572321,
-1.00000000000114));
#8281=CARTESIAN_POINT('',(-21.5938622919806,-0.636266271594385,4.082419099807E-15));
#8282=CARTESIAN_POINT('Origin',(3.64291929955129E-14,-0.121376657232174,
1.));
#8283=CARTESIAN_POINT('',(-14.831751721668,-15.8242152817228,1.));
#8284=CARTESIAN_POINT('',(-14.0664766164573,-16.5132720814551,1.));
#8285=CARTESIAN_POINT('Origin',(4.60655819045641E-12,-0.121376657226993,
1.00000000000115));
#8286=CARTESIAN_POINT('',(-14.831751721668,-15.8242152817229,-0.999999999999996));
#8287=CARTESIAN_POINT('',(-14.831751721668,-15.8242152817229,4.082419099807E-15));
#8288=CARTESIAN_POINT('',(-14.0664766164573,-16.5132720814551,-0.999999999999996));
#8289=CARTESIAN_POINT('Origin',(5.37937749900408E-12,-0.121376657226309,
-1.00000000000114));
#8290=CARTESIAN_POINT('',(-14.0664766164573,-16.5132720814551,4.082419099807E-15));
#8291=CARTESIAN_POINT('Origin',(3.64291929955129E-14,-0.121376657232174,
1.));
#8292=CARTESIAN_POINT('',(-17.7724460902854,-12.3973760042466,-0.999999999999996));
#8293=CARTESIAN_POINT('',(-17.1671570465239,-13.2304849007391,-0.999999999999996));
#8294=CARTESIAN_POINT('Origin',(1.84574577843932E-12,-0.121376657230891,
-1.00000000000114));
#8295=CARTESIAN_POINT('',(-17.1671570465239,-13.2304849007391,1.));
#8296=CARTESIAN_POINT('',(-17.1671570465239,-13.2304849007391,4.082419099807E-15));
#8297=CARTESIAN_POINT('',(-17.7724460902854,-12.3973760042466,1.));
#8298=CARTESIAN_POINT('Origin',(1.84574577843932E-12,-0.121376657230891,
1.00000000000115));
#8299=CARTESIAN_POINT('',(-17.7724460902854,-12.3973760042466,4.082419099807E-15));
#8300=CARTESIAN_POINT('Origin',(3.64291929955129E-14,-0.121376657232174,
1.));
#8301=CARTESIAN_POINT('',(-11.2428386321728,-18.5647651607291,1.));
#8302=CARTESIAN_POINT('',(-10.3510236598078,-19.0796547750914,1.));
#8303=CARTESIAN_POINT('Origin',(9.67975699595058E-13,-0.121376657230781,
1.00000000000115));
#8304=CARTESIAN_POINT('',(-11.2428386321728,-18.5647651607291,-0.999999999999996));
#8305=CARTESIAN_POINT('',(-11.2428386321728,-18.5647651607291,4.082419099807E-15));
#8306=CARTESIAN_POINT('',(-10.3510236598078,-19.0796547750914,-0.999999999999996));
#8307=CARTESIAN_POINT('Origin',(9.67975699595058E-13,-0.121376657230781,
-1.00000000000114));
#8308=CARTESIAN_POINT('',(-10.3510236598078,-19.0796547750914,4.082419099807E-15));
#8309=CARTESIAN_POINT('Origin',(3.64291929955129E-14,-0.121376657232174,
1.));
#8310=CARTESIAN_POINT('',(-7.16255954532629,-20.4992504609354,1.));
#8311=CARTESIAN_POINT('',(-6.18318129950237,-20.8174697430656,1.));
#8312=CARTESIAN_POINT('Origin',(2.8796409701215E-13,-0.121376657232032,
1.00000000000115));
#8313=CARTESIAN_POINT('',(-7.16255954532628,-20.4992504609354,-0.999999999999996));
#8314=CARTESIAN_POINT('',(-7.16255954532628,-20.4992504609354,4.082419099807E-15));
#8315=CARTESIAN_POINT('',(-6.18318129950239,-20.8174697430656,-0.999999999999996));
#8316=CARTESIAN_POINT('Origin',(1.0698907038087E-12,-0.121376657229371,
-1.00000000000114));
#8317=CARTESIAN_POINT('',(-6.18318129950239,-20.8174697430656,4.082419099807E-15));
#8318=CARTESIAN_POINT('Origin',(3.64291929955129E-14,-0.121376657232174,
1.));
#8319=CARTESIAN_POINT('',(-19.936399283099,-8.43401664852542,-0.999999999999996));
#8320=CARTESIAN_POINT('',(-19.5175503364984,-9.37476678530143,-0.999999999999996));
#8321=CARTESIAN_POINT('Origin',(4.32813507256213E-12,-0.12137665723024,
-1.00000000000114));
#8322=CARTESIAN_POINT('',(-19.5175503364984,-9.37476678530144,1.));
#8323=CARTESIAN_POINT('',(-19.5175503364984,-9.37476678530143,4.082419099807E-15));
#8324=CARTESIAN_POINT('',(-19.936399283099,-8.43401664852541,1.));
#8325=CARTESIAN_POINT('Origin',(9.83414738531252E-12,-0.121376657227855,
1.00000000000115));
#8326=CARTESIAN_POINT('',(-19.936399283099,-8.43401664852541,4.082419099807E-15));
#8327=CARTESIAN_POINT('Origin',(3.64291929955129E-14,-0.121376657232174,
1.));
#8328=CARTESIAN_POINT('',(-21.2290361617836,-4.10735503671244,-0.999999999999996));
#8329=CARTESIAN_POINT('',(-21.0149330211704,-5.11463111857488,-0.999999999999996));
#8330=CARTESIAN_POINT('Origin',(6.55378529224038E-12,-0.121376657230702,
-1.00000000000114));
#8331=CARTESIAN_POINT('',(-21.0149330211704,-5.11463111857489,1.));
#8332=CARTESIAN_POINT('',(-21.0149330211704,-5.11463111857488,4.082419099807E-15));
#8333=CARTESIAN_POINT('',(-21.2290361617836,-4.10735503671244,1.));
#8334=CARTESIAN_POINT('Origin',(6.48960052362924E-12,-0.121376657231027,
1.00000000000115));
#8335=CARTESIAN_POINT('',(-21.2290361617836,-4.10735503671244,4.082419099807E-15));
#8336=CARTESIAN_POINT('Origin',(3.64291929955129E-14,-0.121376657232174,
1.));
#8337=CARTESIAN_POINT('',(-21.0149330211704,4.87187780411067,-0.999999999999996));
#8338=CARTESIAN_POINT('',(-21.2290361617835,3.86460172224823,-0.999999999999996));
#8339=CARTESIAN_POINT('Origin',(5.27876353739742E-12,-0.121376657233244,
-1.00000000000114));
#8340=CARTESIAN_POINT('',(-21.2290361617835,3.86460172224823,1.));
#8341=CARTESIAN_POINT('',(-21.2290361617835,3.86460172224823,4.082419099807E-15));
#8342=CARTESIAN_POINT('',(-21.0149330211704,4.87187780411067,1.));
#8343=CARTESIAN_POINT('Origin',(5.9015292652731E-12,-0.12137665723334,1.00000000000115));
#8344=CARTESIAN_POINT('',(-21.0149330211704,4.87187780411067,4.082419099807E-15));
#8345=CARTESIAN_POINT('Origin',(3.64291929955129E-14,-0.121376657232174,
1.));
#8346=CARTESIAN_POINT('',(-10.3510236598076,18.8369014606271,1.));
#8347=CARTESIAN_POINT('',(-11.2428386321727,18.3220118462648,1.));
#8348=CARTESIAN_POINT('Origin',(-3.3506183938492E-12,-0.121376657226028,
1.00000000000115));
#8349=CARTESIAN_POINT('',(-10.3510236598076,18.8369014606271,-0.999999999999996));
#8350=CARTESIAN_POINT('',(-10.3510236598076,18.8369014606271,4.082419099807E-15));
#8351=CARTESIAN_POINT('',(-11.2428386321727,18.3220118462648,-0.999999999999996));
#8352=CARTESIAN_POINT('Origin',(-1.02522157430229E-12,-0.121376657230094,
-1.00000000000114));
#8353=CARTESIAN_POINT('',(-11.2428386321727,18.3220118462648,4.082419099807E-15));
#8354=CARTESIAN_POINT('Origin',(3.64291929955129E-14,-0.121376657232174,
1.));
#8355=CARTESIAN_POINT('',(-14.0664766164572,16.2705187669908,1.));
#8356=CARTESIAN_POINT('',(-14.8317517216679,15.5814619672586,1.));
#8357=CARTESIAN_POINT('Origin',(7.07246761155744E-12,-0.121376657239715,
1.00000000000115));
#8358=CARTESIAN_POINT('',(-14.0664766164572,16.2705187669908,-0.999999999999996));
#8359=CARTESIAN_POINT('',(-14.0664766164572,16.2705187669908,4.082419099807E-15));
#8360=CARTESIAN_POINT('',(-14.8317517216679,15.5814619672586,-0.999999999999996));
#8361=CARTESIAN_POINT('Origin',(2.66019845041043E-12,-0.121376657234943,
-1.00000000000114));
#8362=CARTESIAN_POINT('',(-14.8317517216679,15.5814619672586,4.082419099807E-15));
#8363=CARTESIAN_POINT('Origin',(3.64291929955129E-14,-0.121376657232174,
1.));
#8364=CARTESIAN_POINT('',(-19.5175503364983,9.13201347083722,-0.999999999999996));
#8365=CARTESIAN_POINT('',(-19.936399283099,8.1912633340612,-0.999999999999996));
#8366=CARTESIAN_POINT('Origin',(-5.58060542221739E-12,-0.121376657229723,
-1.00000000000114));
#8367=CARTESIAN_POINT('',(-19.936399283099,8.19126333406119,1.));
#8368=CARTESIAN_POINT('',(-19.936399283099,8.1912633340612,4.082419099807E-15));
#8369=CARTESIAN_POINT('',(-19.5175503364983,9.13201347083722,1.));
#8370=CARTESIAN_POINT('Origin',(1.84921522539128E-12,-0.12137665723286,
1.00000000000115));
#8371=CARTESIAN_POINT('',(-19.5175503364983,9.13201347083722,4.082419099807E-15));
#8372=CARTESIAN_POINT('Origin',(3.64291929955129E-14,-0.121376657232174,
1.));
#8373=CARTESIAN_POINT('',(-17.1671570465239,12.9877315862749,-0.999999999999996));
#8374=CARTESIAN_POINT('',(-17.7724460902853,12.1546226897824,-0.999999999999996));
#8375=CARTESIAN_POINT('Origin',(1.38951350425742E-12,-0.121376657233194,
-1.00000000000114));
#8376=CARTESIAN_POINT('',(-17.7724460902853,12.1546226897824,1.));
#8377=CARTESIAN_POINT('',(-17.7724460902853,12.1546226897824,4.082419099807E-15));
#8378=CARTESIAN_POINT('',(-17.1671570465239,12.9877315862749,1.));
#8379=CARTESIAN_POINT('Origin',(-1.54737334057131E-12,-0.121376657230937,
1.00000000000115));
#8380=CARTESIAN_POINT('',(-17.1671570465239,12.9877315862749,4.082419099807E-15));
#8381=CARTESIAN_POINT('Origin',(3.64291929955129E-14,-0.121376657232174,
1.));
#8382=CARTESIAN_POINT('',(-6.18318129950226,20.5747164286013,-0.999999999999996));
#8383=CARTESIAN_POINT('',(-7.16255954532614,20.2564971464711,-0.999999999999996));
#8384=CARTESIAN_POINT('Origin',(1.00440489259057E-12,-0.121376657234216,
-1.00000000000114));
#8385=CARTESIAN_POINT('',(-7.16255954532614,20.2564971464711,1.));
#8386=CARTESIAN_POINT('',(-7.16255954532614,20.2564971464711,4.082419099807E-15));
#8387=CARTESIAN_POINT('',(-6.18318129950225,20.5747164286013,1.));
#8388=CARTESIAN_POINT('Origin',(-2.04263689296269E-13,-0.121376657230938,
1.00000000000115));
#8389=CARTESIAN_POINT('',(-6.18318129950226,20.5747164286013,4.082419099807E-15));
#8390=CARTESIAN_POINT('Origin',(3.64291929955129E-14,-0.121376657232174,
1.));
#8391=CARTESIAN_POINT('',(-1.74510424621302,21.4080128178516,-0.999999999999996));
#8392=CARTESIAN_POINT('',(-2.7692422365749,21.3003715775681,-0.999999999999996));
#8393=CARTESIAN_POINT('Origin',(1.26483025442159E-12,-0.121376657242586,
-1.00000000000114));
#8394=CARTESIAN_POINT('',(-2.7692422365749,21.3003715775681,1.));
#8395=CARTESIAN_POINT('',(-2.7692422365749,21.3003715775681,4.082419099807E-15));
#8396=CARTESIAN_POINT('',(-1.74510424621301,21.4080128178516,1.));
#8397=CARTESIAN_POINT('Origin',(1.26331237138011E-12,-0.121376657242524,
1.00000000000115));
#8398=CARTESIAN_POINT('',(-1.74510424621302,21.4080128178516,4.082419099807E-15));
#8399=CARTESIAN_POINT('Origin',(3.64291929955129E-14,-0.121376657232174,
1.));
#8400=CARTESIAN_POINT('',(1.74510424621309,21.4080128178516,-0.999999999999996));
#8401=CARTESIAN_POINT('Origin',(-4.11996825544492E-14,-0.121376657231786,
-1.00000000000114));
#8402=CARTESIAN_POINT('',(1.74510424621309,21.4080128178516,1.));
#8403=CARTESIAN_POINT('',(1.74510424621309,21.4080128178516,4.082419099807E-15));
#8404=CARTESIAN_POINT('Origin',(-4.26525134655797E-13,-0.121376657236744,
1.00000000000115));
#8405=CARTESIAN_POINT('Origin',(3.64291929955129E-14,-0.121376657232174,
1.));
#8406=CARTESIAN_POINT('',(6.18318129950261,20.5747164286012,-0.999999999999996));
#8407=CARTESIAN_POINT('Origin',(-7.04297731246584E-13,-0.121376657234403,
-1.00000000000114));
#8408=CARTESIAN_POINT('',(6.18318129950261,20.5747164286012,1.));
#8409=CARTESIAN_POINT('',(6.18318129950261,20.5747164286012,4.082419099807E-15));
#8410=CARTESIAN_POINT('Origin',(5.85469173142172E-13,-0.121376657230185,
1.00000000000115));
#8411=CARTESIAN_POINT('Origin',(3.64291929955129E-14,-0.121376657232174,
1.));
#8412=CARTESIAN_POINT('',(6.18318129950219,-20.8174697430657,1.));
#8413=CARTESIAN_POINT('Origin',(2.9620403352304E-13,-0.121376657232835,
1.00000000000115));
#8414=CARTESIAN_POINT('',(6.18318129950219,-20.8174697430657,-0.999999999999996));
#8415=CARTESIAN_POINT('',(6.18318129950219,-20.8174697430657,4.082419099807E-15));
#8416=CARTESIAN_POINT('Origin',(-8.15753714578094E-13,-0.12137665722947,
-1.00000000000114));
#8417=CARTESIAN_POINT('Origin',(3.64291929955129E-14,-0.121376657232174,
1.));
#8418=CARTESIAN_POINT('',(10.3510236598076,-19.0796547750915,1.));
#8419=CARTESIAN_POINT('',(11.2428386321726,-18.5647651607292,1.));
#8420=CARTESIAN_POINT('Origin',(-7.0082828429463E-13,-0.12137665723075,
1.00000000000115));
#8421=CARTESIAN_POINT('',(10.3510236598076,-19.0796547750915,-0.999999999999996));
#8422=CARTESIAN_POINT('',(10.3510236598076,-19.0796547750915,4.082419099807E-15));
#8423=CARTESIAN_POINT('',(11.2428386321726,-18.5647651607292,-0.999999999999996));
#8424=CARTESIAN_POINT('Origin',(-3.07046055247895E-13,-0.121376657231387,
-1.00000000000114));
#8425=CARTESIAN_POINT('',(11.2428386321726,-18.5647651607292,4.082419099807E-15));
#8426=CARTESIAN_POINT('Origin',(3.64291929955129E-14,-0.121376657232174,
1.));
#8427=CARTESIAN_POINT('',(17.1671570465238,-13.2304849007394,1.));
#8428=CARTESIAN_POINT('',(17.7724460902853,-12.3973760042469,1.));
#8429=CARTESIAN_POINT('Origin',(7.65013052905772E-13,-0.121376657232576,
1.00000000000115));
#8430=CARTESIAN_POINT('',(17.1671570465238,-13.2304849007394,-0.999999999999996));
#8431=CARTESIAN_POINT('',(17.1671570465238,-13.2304849007394,4.082419099807E-15));
#8432=CARTESIAN_POINT('',(17.7724460902853,-12.3973760042469,-0.999999999999996));
#8433=CARTESIAN_POINT('Origin',(-2.69922972861991E-12,-0.121376657230187,
-1.00000000000114));
#8434=CARTESIAN_POINT('',(17.7724460902853,-12.3973760042469,4.082419099807E-15));
#8435=CARTESIAN_POINT('Origin',(3.64291929955129E-14,-0.121376657232174,
1.));
#8436=CARTESIAN_POINT('',(14.0664766164571,-16.5132720814553,-0.999999999999996));
#8437=CARTESIAN_POINT('',(14.8317517216679,-15.8242152817231,-0.999999999999996));
#8438=CARTESIAN_POINT('Origin',(-4.8017145815038E-12,-0.121376657226941,
-1.00000000000114));
#8439=CARTESIAN_POINT('',(14.8317517216679,-15.8242152817231,1.));
#8440=CARTESIAN_POINT('',(14.8317517216679,-15.8242152817231,4.082419099807E-15));
#8441=CARTESIAN_POINT('',(14.0664766164571,-16.5132720814553,1.));
#8442=CARTESIAN_POINT('Origin',(-3.74526798463393E-12,-0.121376657228061,
1.00000000000115));
#8443=CARTESIAN_POINT('',(14.0664766164571,-16.5132720814553,4.082419099807E-15));
#8444=CARTESIAN_POINT('Origin',(3.64291929955129E-14,-0.121376657232174,
1.));
#8445=CARTESIAN_POINT('',(19.5175503364983,-9.37476678530171,1.));
#8446=CARTESIAN_POINT('',(19.936399283099,-8.43401664852567,1.));
#8447=CARTESIAN_POINT('Origin',(-1.16746889933239E-12,-0.121376657231723,
1.00000000000115));
#8448=CARTESIAN_POINT('',(19.5175503364983,-9.37476678530171,-0.999999999999996));
#8449=CARTESIAN_POINT('',(19.5175503364983,-9.37476678530171,4.082419099807E-15));
#8450=CARTESIAN_POINT('',(19.936399283099,-8.43401664852568,-0.999999999999996));
#8451=CARTESIAN_POINT('Origin',(-3.51108031537706E-12,-0.121376657230407,
-1.00000000000114));
#8452=CARTESIAN_POINT('',(19.936399283099,-8.43401664852568,4.082419099807E-15));
#8453=CARTESIAN_POINT('Origin',(3.64291929955129E-14,-0.121376657232174,
1.));
#8454=CARTESIAN_POINT('',(21.0149330211704,-5.11463111857516,1.));
#8455=CARTESIAN_POINT('',(21.2290361617836,-4.10735503671271,1.));
#8456=CARTESIAN_POINT('Origin',(-1.57339419271096E-12,-0.121376657231742,
1.00000000000115));
#8457=CARTESIAN_POINT('',(21.0149330211704,-5.11463111857515,-0.999999999999996));
#8458=CARTESIAN_POINT('',(21.0149330211704,-5.11463111857516,4.082419099807E-15));
#8459=CARTESIAN_POINT('',(21.2290361617836,-4.10735503671272,-0.999999999999996));
#8460=CARTESIAN_POINT('Origin',(-5.76622083414691E-12,-0.121376657230946,
-1.00000000000114));
#8461=CARTESIAN_POINT('',(21.2290361617836,-4.10735503671272,4.082419099807E-15));
#8462=CARTESIAN_POINT('Origin',(3.64291929955129E-14,-0.121376657232174,
1.));
#8463=CARTESIAN_POINT('',(21.5938622919806,-0.636266271594677,1.));
#8464=CARTESIAN_POINT('',(21.5938622919806,0.393512957129885,1.));
#8465=CARTESIAN_POINT('Origin',(2.78770062589473E-12,-0.121376657232179,
1.00000000000115));
#8466=CARTESIAN_POINT('',(21.5938622919806,-0.636266271594671,-0.999999999999996));
#8467=CARTESIAN_POINT('',(21.5938622919806,-0.636266271594672,4.082419099807E-15));
#8468=CARTESIAN_POINT('',(21.5938622919806,0.393512957129885,-0.999999999999996));
#8469=CARTESIAN_POINT('Origin',(2.78770062589473E-12,-0.121376657232179,
-1.00000000000114));
#8470=CARTESIAN_POINT('',(21.5938622919806,0.393512957129885,4.082419099807E-15));
#8471=CARTESIAN_POINT('Origin',(3.64291929955129E-14,-0.121376657232174,
1.));
#8472=CARTESIAN_POINT('',(21.2290361617837,3.86460172224794,1.));
#8473=CARTESIAN_POINT('',(21.0149330211705,4.87187780411038,1.));
#8474=CARTESIAN_POINT('Origin',(3.40526218334247E-12,-0.121376657231491,
1.00000000000115));
#8475=CARTESIAN_POINT('',(21.2290361617837,3.86460172224794,-0.999999999999996));
#8476=CARTESIAN_POINT('',(21.2290361617837,3.86460172224794,4.082419099807E-15));
#8477=CARTESIAN_POINT('',(21.0149330211705,4.87187780411038,-0.999999999999996));
#8478=CARTESIAN_POINT('Origin',(3.37403716077489E-12,-0.121376657231511,
-1.00000000000114));
#8479=CARTESIAN_POINT('',(21.0149330211705,4.87187780411038,4.082419099807E-15));
#8480=CARTESIAN_POINT('Origin',(3.64291929955129E-14,-0.121376657232174,
1.));
#8481=CARTESIAN_POINT('',(14.8317517216682,15.5814619672584,1.));
#8482=CARTESIAN_POINT('',(14.0664766164575,16.2705187669906,1.));
#8483=CARTESIAN_POINT('Origin',(6.18428919185732E-13,-0.121376657231304,
1.00000000000115));
#8484=CARTESIAN_POINT('',(14.8317517216682,15.5814619672584,-0.999999999999996));
#8485=CARTESIAN_POINT('',(14.8317517216682,15.5814619672584,4.082419099807E-15));
#8486=CARTESIAN_POINT('',(14.0664766164575,16.2705187669906,-0.999999999999996));
#8487=CARTESIAN_POINT('Origin',(-4.92227786308419E-12,-0.121376657237505,
-1.00000000000114));
#8488=CARTESIAN_POINT('',(14.0664766164575,16.2705187669906,4.082419099807E-15));
#8489=CARTESIAN_POINT('Origin',(3.64291929955129E-14,-0.121376657232174,
1.));
#8490=CARTESIAN_POINT('',(11.242838632173,18.3220118462647,-0.999999999999996));
#8491=CARTESIAN_POINT('',(10.351023659808,18.836901460627,-0.999999999999996));
#8492=CARTESIAN_POINT('Origin',(-6.7394007041699E-13,-0.12137665723334,
-1.00000000000114));
#8493=CARTESIAN_POINT('',(10.351023659808,18.836901460627,1.));
#8494=CARTESIAN_POINT('',(10.351023659808,18.836901460627,4.082419099807E-15));
#8495=CARTESIAN_POINT('',(11.242838632173,18.3220118462647,1.));
#8496=CARTESIAN_POINT('Origin',(-1.03302782994419E-12,-0.121376657233805,
1.00000000000115));
#8497=CARTESIAN_POINT('',(11.242838632173,18.3220118462647,4.082419099807E-15));
#8498=CARTESIAN_POINT('Origin',(3.64291929955129E-14,-0.121376657232174,
1.));
#8499=CARTESIAN_POINT('',(17.7724460902855,12.1546226897822,-0.999999999999996));
#8500=CARTESIAN_POINT('',(17.1671570465241,12.9877315862747,-0.999999999999996));
#8501=CARTESIAN_POINT('Origin',(-4.61956861652624E-12,-0.121376657235823,
-1.00000000000114));
#8502=CARTESIAN_POINT('',(17.1671570465241,12.9877315862747,1.));
#8503=CARTESIAN_POINT('',(17.1671570465241,12.9877315862747,4.082419099807E-15));
#8504=CARTESIAN_POINT('',(17.7724460902855,12.1546226897822,1.));
#8505=CARTESIAN_POINT('Origin',(-4.1286418728248E-12,-0.121376657235486,
1.00000000000115));
#8506=CARTESIAN_POINT('',(17.7724460902855,12.1546226897822,4.082419099807E-15));
#8507=CARTESIAN_POINT('Origin',(3.64291929955129E-14,-0.121376657232174,
1.));
#8508=CARTESIAN_POINT('',(19.9363992830991,8.19126333406092,-0.999999999999996));
#8509=CARTESIAN_POINT('',(19.5175503364985,9.13201347083695,-0.999999999999996));
#8510=CARTESIAN_POINT('Origin',(-1.92380833485828E-12,-0.121376657233156,
-1.00000000000114));
#8511=CARTESIAN_POINT('',(19.5175503364985,9.13201347083695,1.));
#8512=CARTESIAN_POINT('',(19.5175503364985,9.13201347083695,4.082419099807E-15));
#8513=CARTESIAN_POINT('',(19.9363992830991,8.19126333406092,1.));
#8514=CARTESIAN_POINT('Origin',(-3.03403135948344E-12,-0.121376657233847,
1.00000000000115));
#8515=CARTESIAN_POINT('',(19.9363992830991,8.19126333406092,4.082419099807E-15));
#8516=CARTESIAN_POINT('Origin',(3.64291929955129E-14,-0.121376657232174,
1.));
#8517=CARTESIAN_POINT('',(-2.76924223657505,-21.5431248920325,1.));
#8518=CARTESIAN_POINT('',(-1.74510424621302,-21.650766132316,1.));
#8519=CARTESIAN_POINT('Origin',(-2.18683578190326E-13,-0.121376657234204,
1.00000000000115));
#8520=CARTESIAN_POINT('',(-2.76924223657505,-21.5431248920325,-0.999999999999996));
#8521=CARTESIAN_POINT('',(-2.76924223657505,-21.5431248920325,4.082419099807E-15));
#8522=CARTESIAN_POINT('',(-1.74510424621302,-21.650766132316,-0.999999999999996));
#8523=CARTESIAN_POINT('Origin',(-2.18683578190326E-13,-0.121376657234204,
-1.00000000000114));
#8524=CARTESIAN_POINT('',(-1.74510424621302,-21.650766132316,4.082419099807E-15));
#8525=CARTESIAN_POINT('Origin',(3.55704336920074E-14,-0.121376657232177,
-0.999999999999996));
#8526=CARTESIAN_POINT('',(-13.5539059861829,-13.3451379890505,-0.999999999999996));
#8527=CARTESIAN_POINT('Origin',(-9.43508879143737,-17.0370640084497,-1.00000000000001));
#8528=CARTESIAN_POINT('',(-13.5596392883186,-12.7982291301722,-0.999999999999996));
#8529=CARTESIAN_POINT('Origin',(-13.8554859637001,-13.0748150023091,-0.999999999999996));
#8530=CARTESIAN_POINT('',(-14.024775605964,-12.2816429146937,-0.999999999999996));
#8531=CARTESIAN_POINT('Origin',(-8.74300631892311E-13,-0.121376657233123,
-0.999999999999996));
#8532=CARTESIAN_POINT('',(-14.5680891476276,-12.218773477621,-0.999999999999996));
#8533=CARTESIAN_POINT('Origin',(-14.3307707100941,-12.5469578148565,-0.999999999999996));
#8534=CARTESIAN_POINT('Origin',(-17.8092567781527,-7.73660824112161,-0.999999999999996));
#8535=CARTESIAN_POINT('',(-16.0070951984253,-10.2381515658545,-0.999999999999996));
#8536=CARTESIAN_POINT('Origin',(-12.7458786225912,-14.7057503909453,-1.));
#8537=CARTESIAN_POINT('',(-15.8989944685809,-9.70200195718166,-0.999999999999996));
#8538=CARTESIAN_POINT('Origin',(-16.2458816206227,-9.91103378190783,-0.999999999999996));
#8539=CARTESIAN_POINT('',(-16.2465621281866,-9.09999711167674,-0.999999999999996));
#8540=CARTESIAN_POINT('Origin',(-2.48412401759879E-12,-0.121376657233779,
-0.999999999999996));
#8541=CARTESIAN_POINT('',(-16.7649316744485,-8.92554028555318,-0.999999999999996));
#8542=CARTESIAN_POINT('Origin',(-16.6010325746198,-9.29589428522826,-0.999999999999995));
#8543=CARTESIAN_POINT('Origin',(-19.0033774629777,-3.86744447109249,-1.00000000000001));
#8544=CARTESIAN_POINT('',(-17.7606975399316,-6.68901353347958,-0.999999999999996));
#8545=CARTESIAN_POINT('Origin',(-15.4996123964263,-11.7370296576879,-1.));
#8546=CARTESIAN_POINT('',(-17.5434872987264,-6.18705548564248,-0.999999999999996));
#8547=CARTESIAN_POINT('Origin',(-17.926254294335,-6.31939756917143,-0.999999999999996));
#8548=CARTESIAN_POINT('',(-17.758295925753,-5.52594251059953,-0.999999999999996));
#8549=CARTESIAN_POINT('Origin',(9.73179870022989E-13,-0.121376657231793,
-0.999999999999996));
#8550=CARTESIAN_POINT('',(-18.2290662400285,-5.24752289586338,-0.999999999999996));
#8551=CARTESIAN_POINT('Origin',(-18.1457496550421,-5.64386031103663,-0.999999999999996));
#8552=CARTESIAN_POINT('Origin',(-19.3669593643481,0.165440438030001,-1.));
#8553=CARTESIAN_POINT('',(-18.7380721736606,-2.85283825459442,-0.999999999999996));
#8554=CARTESIAN_POINT('Origin',(-17.5759387331454,-8.26064915022346,-0.999999999999996));
#8555=CARTESIAN_POINT('',(-18.4212455509255,-2.40700974294545,-0.999999999999996));
#8556=CARTESIAN_POINT('Origin',(-18.8231636356729,-2.45687810117919,-0.999999999999995));
#8557=CARTESIAN_POINT('',(-18.4939069776057,-1.71568244774586,-0.999999999999996));
#8558=CARTESIAN_POINT('Origin',(3.52669282666085E-12,-0.121376657231728,
-0.999999999999996));
#8559=CARTESIAN_POINT('',(-18.8965031381544,-1.34546831756664,-0.999999999999996));
#8560=CARTESIAN_POINT('Origin',(-18.8974104025717,-1.75046730135707,-0.999999999999995));
#8561=CARTESIAN_POINT('Origin',(-18.8841122085148,4.18579006378843,-1.));
#8562=CARTESIAN_POINT('',(-18.8965031381544,1.10271500310242,-0.999999999999996));
#8563=CARTESIAN_POINT('Origin',(-18.8841122085149,-4.42854337825268,-0.999999999999996));
#8564=CARTESIAN_POINT('',(-18.4939069776057,1.47292913328164,-0.999999999999996));
#8565=CARTESIAN_POINT('Origin',(-18.8974104025716,1.50771398689285,-0.999999999999996));
#8566=CARTESIAN_POINT('',(-18.4212455509255,2.16425642848123,-0.999999999999996));
#8567=CARTESIAN_POINT('Origin',(-3.32199545649559E-12,-0.121376657231894,
-0.999999999999996));
#8568=CARTESIAN_POINT('',(-18.7380721736606,2.61008494013019,-0.999999999999996));
#8569=CARTESIAN_POINT('Origin',(-18.8231636356729,2.21412478671497,-0.999999999999996));
#8570=CARTESIAN_POINT('Origin',(-17.5759387331454,8.01789583575931,-1.00000000000001));
#8571=CARTESIAN_POINT('',(-18.2290662400284,5.00476958139915,-0.999999999999996));
#8572=CARTESIAN_POINT('Origin',(-19.3669593643482,-0.408193752494279,-1.00000000000001));
#8573=CARTESIAN_POINT('',(-17.7582959257529,5.2831891961353,-0.999999999999996));
#8574=CARTESIAN_POINT('Origin',(-18.1457496550421,5.40110699657241,-0.999999999999996));
#8575=CARTESIAN_POINT('',(-17.5434872987263,5.94430217117825,-0.999999999999996));
#8576=CARTESIAN_POINT('Origin',(7.0082828429463E-13,-0.121376657232305,
-0.999999999999996));
#8577=CARTESIAN_POINT('',(-17.7606975399316,6.44626021901535,-0.999999999999996));
#8578=CARTESIAN_POINT('Origin',(-17.9262542943349,6.0766442547072,-0.999999999999996));
#8579=CARTESIAN_POINT('Origin',(-15.4996123964262,11.4942763432237,-1.00000000000001));
#8580=CARTESIAN_POINT('',(-16.7649316744485,8.68278697108894,-0.999999999999996));
#8581=CARTESIAN_POINT('Origin',(-19.0033774629776,3.62469115662824,-1.00000000000001));
#8582=CARTESIAN_POINT('',(-16.2465621281866,8.85724379721251,-0.999999999999996));
#8583=CARTESIAN_POINT('Origin',(-16.6010325746197,9.05314097076402,-0.999999999999996));
#8584=CARTESIAN_POINT('',(-15.8989944685809,9.45924864271742,-0.999999999999996));
#8585=CARTESIAN_POINT('Origin',(3.8372083288607E-12,-0.121376657234332,
-0.999999999999996));
#8586=CARTESIAN_POINT('',(-16.0070951984252,9.99539825139022,-0.999999999999996));
#8587=CARTESIAN_POINT('Origin',(-16.2458816206226,9.66828046744359,-0.999999999999996));
#8588=CARTESIAN_POINT('Origin',(-12.7458786225911,14.462997076481,-1.));
#8589=CARTESIAN_POINT('',(-14.5680891476275,11.9760201631568,-0.999999999999996));
#8590=CARTESIAN_POINT('Origin',(-17.8092567781527,7.49385492665739,-1.00000000000001));
#8591=CARTESIAN_POINT('',(-14.0247756059639,12.0388896002294,-0.999999999999996));
#8592=CARTESIAN_POINT('Origin',(-14.330770710094,12.3042045003922,-0.999999999999996));
#8593=CARTESIAN_POINT('',(-13.5596392883185,12.555475815708,-0.999999999999996));
#8594=CARTESIAN_POINT('Origin',(1.06442632485937E-11,-0.1213766572417,-0.999999999999996));
#8595=CARTESIAN_POINT('',(-13.5539059861829,13.1023846745862,-0.999999999999996));
#8596=CARTESIAN_POINT('Origin',(-13.8554859637,12.8320616878448,-0.999999999999995));
#8597=CARTESIAN_POINT('Origin',(-9.43508879143732,16.7943106939854,-1.));
#8598=CARTESIAN_POINT('',(-11.7345512196076,14.7405390644231,-0.999999999999996));
#8599=CARTESIAN_POINT('Origin',(-15.8367861138271,11.030196534535,-1.00000000000001));
#8600=CARTESIAN_POINT('',(-11.1900390914206,14.6890734163638,-0.999999999999996));
#8601=CARTESIAN_POINT('Origin',(-11.4341853988698,15.0122105088786,-0.999999999999996));
#8602=CARTESIAN_POINT('',(-10.6276628047883,15.0976637053439,-0.999999999999996));
#8603=CARTESIAN_POINT('Origin',(-9.26342336171615E-13,-0.121376657230733,
-0.999999999999996));
#8604=CARTESIAN_POINT('',(-10.5083460434875,15.6314292729347,-0.999999999999996));
#8605=CARTESIAN_POINT('Origin',(-10.8595390841655,15.4297154950728,-0.999999999999996));
#8606=CARTESIAN_POINT('Origin',(-5.71194030551858,18.3863276037679,-1.));
#8607=CARTESIAN_POINT('',(-8.38815709466669,16.8555209332692,-0.999999999999996));
#8608=CARTESIAN_POINT('Origin',(-13.1721719029961,14.0791608827473,-1.00000000000001));
#8609=CARTESIAN_POINT('',(-7.8662441728172,16.6919694958576,-0.999999999999996));
#8610=CARTESIAN_POINT('Origin',(-8.03787131840593,17.0588061391977,-0.999999999999996));
#8611=CARTESIAN_POINT('',(-7.23120645950465,16.9747065020771,-0.999999999999996));
#8612=CARTESIAN_POINT('Origin',(5.46524631106493E-12,-0.12137665724324,
-0.999999999999996));
#8613=CARTESIAN_POINT('',(-7.0035209540528,17.4720006617854,-0.999999999999996));
#8614=CARTESIAN_POINT('Origin',(-7.38897823680293,17.3477119528257,-0.999999999999996));
#8615=CARTESIAN_POINT('Origin',(-1.73915261931814,19.1694690275264,-0.999999999999996));
#8616=CARTESIAN_POINT('',(-4.67516025384538,18.2285309132174,-0.999999999999996));
#8617=CARTESIAN_POINT('Origin',(-9.93187057291064,16.5074935987233,-0.999999999999996));
#8618=CARTESIAN_POINT('',(-4.19865663743425,17.9600416690753,-0.999999999999996));
#8619=CARTESIAN_POINT('Origin',(-4.29026369134191,18.3545453416493,-0.999999999999996));
#8620=CARTESIAN_POINT('',(-3.51871169276225,18.1045684286397,-0.999999999999996));
#8621=CARTESIAN_POINT('Origin',(1.46844342241437E-12,-0.121376657238497,
-0.999999999999996));
#8622=CARTESIAN_POINT('',(-3.19260839230391,18.5436570394042,-0.999999999999996));
#8623=CARTESIAN_POINT('Origin',(-3.5954835842407,18.5022254123315,-0.999999999999996));
#8624=CARTESIAN_POINT('Origin',(2.30964438172666,19.109507927113,-1.));
#8625=CARTESIAN_POINT('',(-0.757836476023246,18.7995618797112,-0.999999999999996));
#8626=CARTESIAN_POINT('Origin',(-6.25749884038649,18.2090648903413,-1.00000000000001));
#8627=CARTESIAN_POINT('',(-0.347567659605682,18.4378690971619,-0.999999999999996));
#8628=CARTESIAN_POINT('Origin',(-0.35515095399708,18.8427980954396,-0.999999999999996));
#8629=CARTESIAN_POINT('',(0.347567659605759,18.4378690971619,-0.999999999999996));
#8630=CARTESIAN_POINT('Origin',(3.74591850593742E-14,-0.121376657224663,
-0.999999999999996));
#8631=CARTESIAN_POINT('',(0.757836476023318,18.7995618797112,-0.999999999999996));
#8632=CARTESIAN_POINT('Origin',(0.35515095399715,18.8427980954396,-0.999999999999996));
#8633=CARTESIAN_POINT('Origin',(6.25749884038657,18.2090648903413,-1.00000000000001));
#8634=CARTESIAN_POINT('',(4.19865663743457,17.9600416690753,-0.999999999999996));
#8635=CARTESIAN_POINT('Origin',(-1.20715069884536E-12,-0.121376657237335,
-0.999999999999996));
#8636=CARTESIAN_POINT('',(4.6751602538457,18.2285309132174,-0.999999999999996));
#8637=CARTESIAN_POINT('Origin',(4.29026369134224,18.3545453416493,-0.999999999999996));
#8638=CARTESIAN_POINT('Origin',(9.93187057291089,16.5074935987231,-1.));
#8639=CARTESIAN_POINT('',(7.8662441728175,16.6919694958575,-0.999999999999996));
#8640=CARTESIAN_POINT('Origin',(-4.48686227061401E-12,-0.121376657241696,
-0.999999999999996));
#8641=CARTESIAN_POINT('',(8.38815709466699,16.8555209332691,-0.999999999999996));
#8642=CARTESIAN_POINT('Origin',(8.03787131840625,17.0588061391976,-0.999999999999996));
#8643=CARTESIAN_POINT('Origin',(13.1721719029964,14.0791608827472,-1.));
#8644=CARTESIAN_POINT('Origin',(5.71194030551892,18.3863276037678,-1.00000000000001));
#8645=CARTESIAN_POINT('',(11.1900390914209,14.6890734163636,-0.999999999999996));
#8646=CARTESIAN_POINT('Origin',(2.03656536079677E-12,-0.121376657229092,
-0.999999999999996));
#8647=CARTESIAN_POINT('',(11.7345512196078,14.740539064423,-0.999999999999996));
#8648=CARTESIAN_POINT('Origin',(11.4341853988701,15.0122105088784,-0.999999999999996));
#8649=CARTESIAN_POINT('Origin',(15.8367861138273,11.0301965345349,-0.999999999999996));
#8650=CARTESIAN_POINT('Origin',(9.43508879143763,16.7943106939853,-1.));
#8651=CARTESIAN_POINT('',(14.0247756059641,12.0388896002292,-0.999999999999996));
#8652=CARTESIAN_POINT('Origin',(-1.08160008727154E-12,-0.121376657233035,
-0.999999999999996));
#8653=CARTESIAN_POINT('',(14.5680891476277,11.9760201631566,-0.999999999999996));
#8654=CARTESIAN_POINT('Origin',(14.3307707100943,12.304204500392,-0.999999999999996));
#8655=CARTESIAN_POINT('Origin',(17.8092567781528,7.49385492665722,-0.999999999999996));
#8656=CARTESIAN_POINT('Origin',(12.7458786225913,14.4629970764809,-1.00000000000001));
#8657=CARTESIAN_POINT('',(16.2465621281868,8.85724379721227,-0.999999999999996));
#8658=CARTESIAN_POINT('Origin',(-2.16666962149503E-12,-0.121376657233593,
-0.999999999999996));
#8659=CARTESIAN_POINT('',(16.7649316744487,8.68278697108871,-0.999999999999996));
#8660=CARTESIAN_POINT('Origin',(16.6010325746199,9.05314097076378,-0.999999999999996));
#8661=CARTESIAN_POINT('Origin',(19.0033774629777,3.62469115662801,-1.00000000000001));
#8662=CARTESIAN_POINT('Origin',(15.4996123964264,11.4942763432235,-0.999999999999996));
#8663=CARTESIAN_POINT('',(17.7582959257531,5.28318919613505,-0.999999999999996));
#8664=CARTESIAN_POINT('Origin',(-2.30544749957318E-12,-0.121376657233087,
-0.999999999999996));
#8665=CARTESIAN_POINT('',(18.2290662400286,5.0047695813989,-0.999999999999996));
#8666=CARTESIAN_POINT('Origin',(18.1457496550422,5.40110699657215,-0.999999999999995));
#8667=CARTESIAN_POINT('Origin',(19.3669593643482,-0.408193752494484,-1.));
#8668=CARTESIAN_POINT('Origin',(17.5759387331456,8.01789583575902,-1.));
#8669=CARTESIAN_POINT('',(18.4939069776058,1.47292913328138,-0.999999999999996));
#8670=CARTESIAN_POINT('Origin',(-4.20843915271973E-12,-0.121376657232797,
-0.999999999999996));
#8671=CARTESIAN_POINT('',(18.8965031381544,1.10271500310216,-0.999999999999996));
#8672=CARTESIAN_POINT('Origin',(18.8974104025717,1.50771398689259,-0.999999999999996));
#8673=CARTESIAN_POINT('Origin',(18.8841122085149,-4.42854337825293,-1.));
#8674=CARTESIAN_POINT('',(18.8965031381544,-1.34546831756689,-0.999999999999996));
#8675=CARTESIAN_POINT('Origin',(18.884112208515,4.18579006378818,-1.));
#8676=CARTESIAN_POINT('',(18.4939069776058,-1.71568244774611,-0.999999999999996));
#8677=CARTESIAN_POINT('Origin',(18.8974104025717,-1.75046730135732,-0.999999999999996));
#8678=CARTESIAN_POINT('Origin',(-1.14006026841196E-11,-0.121376657231028,
-0.999999999999996));
#8679=CARTESIAN_POINT('Origin',(17.5759387331454,-8.26064915022374,-0.999999999999996));
#8680=CARTESIAN_POINT('',(18.2290662400285,-5.24752289586362,-0.999999999999996));
#8681=CARTESIAN_POINT('Origin',(19.3669593643482,0.165440438029741,-1.00000000000001));
#8682=CARTESIAN_POINT('',(17.758295925753,-5.52594251059977,-0.999999999999996));
#8683=CARTESIAN_POINT('Origin',(18.1457496550421,-5.64386031103686,-0.999999999999996));
#8684=CARTESIAN_POINT('Origin',(-7.66747776381749E-12,-0.121376657229412,
-0.999999999999996));
#8685=CARTESIAN_POINT('Origin',(15.4996123964262,-11.7370296576882,-1.00000000000001));
#8686=CARTESIAN_POINT('',(16.7649316744485,-8.92554028555341,-0.999999999999996));
#8687=CARTESIAN_POINT('Origin',(19.0033774629777,-3.86744447109281,-1.));
#8688=CARTESIAN_POINT('',(16.2465621281866,-9.09999711167697,-0.999999999999996));
#8689=CARTESIAN_POINT('Origin',(16.6010325746197,-9.29589428522849,-0.999999999999996));
#8690=CARTESIAN_POINT('Origin',(-5.0636578263763E-12,-0.121376657229021,
-0.999999999999996));
#8691=CARTESIAN_POINT('Origin',(12.7458786225911,-14.7057503909454,-1.));
#8692=CARTESIAN_POINT('',(14.5680891476275,-12.2187734776212,-0.999999999999996));
#8693=CARTESIAN_POINT('Origin',(17.8092567781527,-7.73660824112183,-1.00000000000001));
#8694=CARTESIAN_POINT('',(14.0247756059639,-12.2816429146939,-0.999999999999996));
#8695=CARTESIAN_POINT('Origin',(14.330770710094,-12.5469578148567,-0.999999999999996));
#8696=CARTESIAN_POINT('Origin',(2.40519409944184E-12,-0.121376657234426,
-0.999999999999996));
#8697=CARTESIAN_POINT('Origin',(9.43508879143727,-17.0370640084498,-0.999999999999996));
#8698=CARTESIAN_POINT('',(11.7345512196075,-14.9832923788876,-0.999999999999996));
#8699=CARTESIAN_POINT('Origin',(15.836786113827,-11.2729498489996,-1.00000000000001));
#8700=CARTESIAN_POINT('',(11.1900390914206,-14.9318267308282,-0.999999999999996));
#8701=CARTESIAN_POINT('Origin',(11.4341853988697,-15.254963823343,-0.999999999999996));
#8702=CARTESIAN_POINT('Origin',(1.15619319673854E-12,-0.121376657233852,
-0.999999999999996));
#8703=CARTESIAN_POINT('Origin',(5.71194030551854,-18.6290809182323,-1.));
#8704=CARTESIAN_POINT('',(8.38815709466665,-17.0982742477336,-0.999999999999996));
#8705=CARTESIAN_POINT('Origin',(13.172171902996,-14.3219141972119,-1.));
#8706=CARTESIAN_POINT('',(7.86624417281716,-16.934722810322,-0.999999999999996));
#8707=CARTESIAN_POINT('Origin',(8.03787131840589,-17.3015594536621,-0.999999999999996));
#8708=CARTESIAN_POINT('Origin',(-4.28953747522165E-12,-0.121376657222038,
-0.999999999999996));
#8709=CARTESIAN_POINT('',(4.67516025384533,-18.4712842276818,-0.999999999999996));
#8710=CARTESIAN_POINT('Origin',(9.93187057291061,-16.7502469131877,-1.00000000000001));
#8711=CARTESIAN_POINT('',(4.1986566374342,-18.2027949835397,-0.999999999999996));
#8712=CARTESIAN_POINT('Origin',(4.29026369134186,-18.5972986561137,-0.999999999999996));
#8713=CARTESIAN_POINT('Origin',(2.61075883134509E-13,-0.121376657233687,
-0.999999999999996));
#8714=CARTESIAN_POINT('',(1.74510424621309,-21.650766132316,-0.999999999999996));
#8715=CARTESIAN_POINT('Origin',(-2.82976767018717E-13,-0.121376657227844,
-1.00000000000114));
#8716=CARTESIAN_POINT('',(0.757836476023318,-19.0423151941755,-0.999999999999996));
#8717=CARTESIAN_POINT('Origin',(6.25749884038654,-18.4518182048057,-1.));
#8718=CARTESIAN_POINT('',(0.347567659605753,-18.6806224116263,-0.999999999999996));
#8719=CARTESIAN_POINT('Origin',(0.355150953997144,-19.085551409904,-0.999999999999996));
#8720=CARTESIAN_POINT('',(-0.347567659605688,-18.6806224116263,-0.999999999999996));
#8721=CARTESIAN_POINT('Origin',(4.2148359455374E-14,-0.12137665722483,-0.999999999999996));
#8722=CARTESIAN_POINT('',(-0.757836476023246,-19.0423151941755,-0.999999999999996));
#8723=CARTESIAN_POINT('Origin',(-0.355150953997086,-19.085551409904,-0.999999999999996));
#8724=CARTESIAN_POINT('Origin',(-6.25749884038644,-18.4518182048057,-1.));
#8725=CARTESIAN_POINT('',(-3.19260839230403,-18.7864103538685,-0.999999999999996));
#8726=CARTESIAN_POINT('Origin',(2.30964438172655,-19.3522612415774,-1.));
#8727=CARTESIAN_POINT('',(-3.51871169276238,-18.3473217431041,-0.999999999999996));
#8728=CARTESIAN_POINT('Origin',(-3.59548358424083,-18.7449787267958,-0.999999999999996));
#8729=CARTESIAN_POINT('',(-4.19865663743438,-18.2027949835397,-0.999999999999996));
#8730=CARTESIAN_POINT('Origin',(1.19327291103755E-12,-0.121376657226644,
-0.999999999999996));
#8731=CARTESIAN_POINT('',(-4.6751602538455,-18.4712842276817,-0.999999999999996));
#8732=CARTESIAN_POINT('Origin',(-4.29026369134204,-18.5972986561136,-0.999999999999996));
#8733=CARTESIAN_POINT('Origin',(-9.93187057291073,-16.7502469131876,-1.));
#8734=CARTESIAN_POINT('',(-7.00352095405292,-17.7147539762497,-0.999999999999996));
#8735=CARTESIAN_POINT('Origin',(-1.73915261931825,-19.4122223419907,-1.));
#8736=CARTESIAN_POINT('',(-7.23120645950477,-17.2174598165414,-0.999999999999996));
#8737=CARTESIAN_POINT('Origin',(-7.38897823680306,-17.59046526729,-0.999999999999996));
#8738=CARTESIAN_POINT('',(-7.86624417281732,-16.9347228103219,-0.999999999999996));
#8739=CARTESIAN_POINT('Origin',(4.03409944338406E-12,-0.121376657223046,
-0.999999999999996));
#8740=CARTESIAN_POINT('',(-8.38815709466681,-17.0982742477335,-0.999999999999996));
#8741=CARTESIAN_POINT('Origin',(-8.03787131840607,-17.301559453662,-0.999999999999995));
#8742=CARTESIAN_POINT('Origin',(-13.1721719029961,-14.3219141972117,-0.999999999999996));
#8743=CARTESIAN_POINT('',(-10.5083460434876,-15.874182587399,-0.999999999999996));
#8744=CARTESIAN_POINT('Origin',(-5.7119403055187,-18.6290809182322,-0.999999999999996));
#8745=CARTESIAN_POINT('',(-10.6276628047884,-15.3404170198082,-0.999999999999996));
#8746=CARTESIAN_POINT('Origin',(-10.8595390841656,-15.6724688095371,-0.999999999999996));
#8747=CARTESIAN_POINT('',(-11.1900390914207,-14.931826730828,-0.999999999999996));
#8748=CARTESIAN_POINT('Origin',(6.0281640790194E-13,-0.121376657231363,
-0.999999999999996));
#8749=CARTESIAN_POINT('',(-11.7345512196077,-14.9832923788874,-0.999999999999996));
#8750=CARTESIAN_POINT('Origin',(-11.4341853988699,-15.2549638233429,-0.999999999999995));
#8751=CARTESIAN_POINT('Origin',(-15.8367861138271,-11.2729498489993,-1.));
#8752=CARTESIAN_POINT('',(1.49999999999993,5.62862334276781,-0.999999999999996));
#8753=CARTESIAN_POINT('',(-1.49999999999993,5.62862334276781,-0.999999999999996));
#8754=CARTESIAN_POINT('',(3.55704336920074E-14,5.62862334276781,-0.999999999999996));
#8755=CARTESIAN_POINT('',(-1.49999999999993,-0.121376657232177,-0.999999999999996));
#8756=CARTESIAN_POINT('',(1.49999999999993,-0.121376657232177,-0.999999999999996));
#8757=CARTESIAN_POINT('Origin',(3.55704336920074E-14,-0.121376657232177,
1.));
#8758=CARTESIAN_POINT('',(-13.5539059861829,-13.3451379890505,1.));
#8759=CARTESIAN_POINT('Origin',(-9.43508879143742,-17.0370640084497,1.00000000000001));
#8760=CARTESIAN_POINT('',(-11.7345512196077,-14.9832923788874,1.));
#8761=CARTESIAN_POINT('Origin',(-15.8367861138271,-11.2729498489993,1.00000000000001));
#8762=CARTESIAN_POINT('',(-11.1900390914207,-14.931826730828,1.));
#8763=CARTESIAN_POINT('Origin',(-11.4341853988699,-15.2549638233429,1.));
#8764=CARTESIAN_POINT('',(-10.6276628047884,-15.3404170198082,1.));
#8765=CARTESIAN_POINT('Origin',(6.0281640790194E-13,-0.121376657231363,
1.));
#8766=CARTESIAN_POINT('',(-10.5083460434876,-15.874182587399,1.));
#8767=CARTESIAN_POINT('Origin',(-10.8595390841656,-15.6724688095371,1.));
#8768=CARTESIAN_POINT('Origin',(-5.7119403055187,-18.6290809182322,1.00000000000001));
#8769=CARTESIAN_POINT('',(-8.38815709466681,-17.0982742477335,1.));
#8770=CARTESIAN_POINT('Origin',(-13.1721719029961,-14.3219141972117,1.));
#8771=CARTESIAN_POINT('',(-7.86624417281732,-16.9347228103219,1.));
#8772=CARTESIAN_POINT('Origin',(-8.03787131840606,-17.301559453662,1.));
#8773=CARTESIAN_POINT('',(-7.23120645950477,-17.2174598165414,1.));
#8774=CARTESIAN_POINT('Origin',(4.03409944338406E-12,-0.121376657223046,
1.));
#8775=CARTESIAN_POINT('',(-7.00352095405292,-17.7147539762497,1.));
#8776=CARTESIAN_POINT('Origin',(-7.38897823680306,-17.59046526729,1.));
#8777=CARTESIAN_POINT('Origin',(-1.73915261931826,-19.4122223419907,1.));
#8778=CARTESIAN_POINT('',(-4.6751602538455,-18.4712842276817,1.));
#8779=CARTESIAN_POINT('Origin',(-9.93187057291071,-16.7502469131876,1.00000000000001));
#8780=CARTESIAN_POINT('',(-4.19865663743438,-18.2027949835397,1.));
#8781=CARTESIAN_POINT('Origin',(-4.29026369134204,-18.5972986561136,1.));
#8782=CARTESIAN_POINT('',(-3.51871169276238,-18.3473217431041,1.));
#8783=CARTESIAN_POINT('Origin',(1.19327291103755E-12,-0.121376657226644,
1.));
#8784=CARTESIAN_POINT('',(-3.19260839230403,-18.7864103538685,1.));
#8785=CARTESIAN_POINT('Origin',(-3.59548358424083,-18.7449787267958,1.));
#8786=CARTESIAN_POINT('Origin',(2.30964438172659,-19.3522612415774,1.00000000000001));
#8787=CARTESIAN_POINT('',(-0.757836476023246,-19.0423151941755,1.));
#8788=CARTESIAN_POINT('Origin',(-6.25749884038647,-18.4518182048057,1.00000000000001));
#8789=CARTESIAN_POINT('',(-0.347567659605688,-18.6806224116263,1.));
#8790=CARTESIAN_POINT('Origin',(-0.355150953997085,-19.085551409904,1.));
#8791=CARTESIAN_POINT('',(0.347567659605753,-18.6806224116263,1.));
#8792=CARTESIAN_POINT('Origin',(4.2148359455374E-14,-0.12137665722483,1.));
#8793=CARTESIAN_POINT('',(0.757836476023318,-19.0423151941755,1.));
#8794=CARTESIAN_POINT('Origin',(0.355150953997144,-19.085551409904,1.));
#8795=CARTESIAN_POINT('',(1.74510424621308,-21.650766132316,1.));
#8796=CARTESIAN_POINT('Origin',(6.25749884038654,-18.4518182048057,1.));
#8797=CARTESIAN_POINT('Origin',(4.24356730310826E-13,-0.121376657236306,
1.00000000000115));
#8798=CARTESIAN_POINT('',(4.1986566374342,-18.2027949835397,1.));
#8799=CARTESIAN_POINT('Origin',(2.61075883134509E-13,-0.121376657233687,
1.));
#8800=CARTESIAN_POINT('',(4.67516025384533,-18.4712842276818,1.));
#8801=CARTESIAN_POINT('Origin',(4.29026369134186,-18.5972986561137,1.));
#8802=CARTESIAN_POINT('Origin',(9.93187057291057,-16.7502469131877,1.00000000000001));
#8803=CARTESIAN_POINT('',(7.86624417281716,-16.934722810322,1.));
#8804=CARTESIAN_POINT('Origin',(-4.28953747522165E-12,-0.121376657222038,
1.));
#8805=CARTESIAN_POINT('',(8.38815709466665,-17.0982742477336,1.));
#8806=CARTESIAN_POINT('Origin',(8.03787131840589,-17.3015594536621,1.));
#8807=CARTESIAN_POINT('Origin',(13.172171902996,-14.3219141972118,1.00000000000001));
#8808=CARTESIAN_POINT('Origin',(5.7119403055185,-18.6290809182323,1.00000000000001));
#8809=CARTESIAN_POINT('',(11.1900390914206,-14.9318267308282,1.));
#8810=CARTESIAN_POINT('Origin',(1.15619319673854E-12,-0.121376657233852,
1.));
#8811=CARTESIAN_POINT('',(11.7345512196075,-14.9832923788876,1.));
#8812=CARTESIAN_POINT('Origin',(11.4341853988697,-15.254963823343,1.));
#8813=CARTESIAN_POINT('Origin',(15.836786113827,-11.2729498489996,1.00000000000001));
#8814=CARTESIAN_POINT('Origin',(9.43508879143727,-17.0370640084498,1.));
#8815=CARTESIAN_POINT('',(14.0247756059639,-12.2816429146939,1.));
#8816=CARTESIAN_POINT('Origin',(2.40519409944184E-12,-0.121376657234426,
1.));
#8817=CARTESIAN_POINT('',(14.5680891476275,-12.2187734776212,1.));
#8818=CARTESIAN_POINT('Origin',(14.330770710094,-12.5469578148567,1.));
#8819=CARTESIAN_POINT('Origin',(17.8092567781528,-7.73660824112176,1.00000000000001));
#8820=CARTESIAN_POINT('Origin',(12.745878622591,-14.7057503909455,1.00000000000001));
#8821=CARTESIAN_POINT('',(16.2465621281866,-9.09999711167697,1.));
#8822=CARTESIAN_POINT('Origin',(-5.0636578263763E-12,-0.121376657229021,
1.));
#8823=CARTESIAN_POINT('',(16.7649316744485,-8.92554028555341,1.));
#8824=CARTESIAN_POINT('Origin',(16.6010325746197,-9.29589428522849,1.));
#8825=CARTESIAN_POINT('Origin',(19.0033774629777,-3.86744447109278,1.00000000000001));
#8826=CARTESIAN_POINT('Origin',(15.4996123964262,-11.7370296576882,1.00000000000001));
#8827=CARTESIAN_POINT('',(17.758295925753,-5.52594251059977,1.));
#8828=CARTESIAN_POINT('Origin',(-7.66747776381749E-12,-0.121376657229412,
1.));
#8829=CARTESIAN_POINT('',(18.2290662400285,-5.24752289586362,1.));
#8830=CARTESIAN_POINT('Origin',(18.1457496550421,-5.64386031103686,1.));
#8831=CARTESIAN_POINT('Origin',(19.3669593643482,0.16544043802976,1.00000000000001));
#8832=CARTESIAN_POINT('Origin',(17.5759387331454,-8.26064915022377,1.00000000000001));
#8833=CARTESIAN_POINT('',(18.4939069776058,-1.71568244774611,1.));
#8834=CARTESIAN_POINT('Origin',(-1.14006026841196E-11,-0.121376657231028,
1.));
#8835=CARTESIAN_POINT('',(18.8965031381544,-1.34546831756689,1.));
#8836=CARTESIAN_POINT('Origin',(18.8974104025717,-1.75046730135732,1.));
#8837=CARTESIAN_POINT('Origin',(18.884112208515,4.18579006378822,1.00000000000001));
#8838=CARTESIAN_POINT('',(18.8965031381544,1.10271500310216,1.));
#8839=CARTESIAN_POINT('Origin',(18.8841122085149,-4.42854337825293,1.00000000000001));
#8840=CARTESIAN_POINT('',(18.4939069776058,1.47292913328138,1.));
#8841=CARTESIAN_POINT('Origin',(18.8974104025717,1.50771398689259,1.));
#8842=CARTESIAN_POINT('Origin',(-4.20843915271973E-12,-0.121376657232797,
1.));
#8843=CARTESIAN_POINT('Origin',(17.5759387331456,8.01789583575901,1.00000000000001));
#8844=CARTESIAN_POINT('',(18.2290662400286,5.0047695813989,1.));
#8845=CARTESIAN_POINT('Origin',(19.3669593643482,-0.408193752494475,1.00000000000001));
#8846=CARTESIAN_POINT('',(17.7582959257531,5.28318919613505,1.));
#8847=CARTESIAN_POINT('Origin',(18.1457496550422,5.40110699657215,1.));
#8848=CARTESIAN_POINT('Origin',(-2.30544749957318E-12,-0.121376657233087,
1.));
#8849=CARTESIAN_POINT('Origin',(15.4996123964264,11.4942763432235,1.));
#8850=CARTESIAN_POINT('',(16.7649316744487,8.68278697108871,1.));
#8851=CARTESIAN_POINT('Origin',(19.0033774629777,3.62469115662802,1.00000000000001));
#8852=CARTESIAN_POINT('',(16.2465621281868,8.85724379721227,1.));
#8853=CARTESIAN_POINT('Origin',(16.6010325746199,9.05314097076379,1.));
#8854=CARTESIAN_POINT('Origin',(-2.16666962149503E-12,-0.121376657233593,
1.));
#8855=CARTESIAN_POINT('Origin',(12.7458786225913,14.4629970764809,1.00000000000001));
#8856=CARTESIAN_POINT('',(14.5680891476277,11.9760201631566,1.));
#8857=CARTESIAN_POINT('Origin',(17.8092567781529,7.49385492665713,1.00000000000001));
#8858=CARTESIAN_POINT('',(14.0247756059641,12.0388896002292,1.));
#8859=CARTESIAN_POINT('Origin',(14.3307707100943,12.304204500392,1.));
#8860=CARTESIAN_POINT('Origin',(-1.08160008727154E-12,-0.121376657233035,
1.));
#8861=CARTESIAN_POINT('Origin',(9.43508879143764,16.7943106939852,1.00000000000001));
#8862=CARTESIAN_POINT('',(11.7345512196078,14.740539064423,1.));
#8863=CARTESIAN_POINT('Origin',(15.8367861138273,11.0301965345349,1.00000000000001));
#8864=CARTESIAN_POINT('',(11.1900390914209,14.6890734163636,1.));
#8865=CARTESIAN_POINT('Origin',(11.4341853988701,15.0122105088784,1.));
#8866=CARTESIAN_POINT('Origin',(2.03656536079677E-12,-0.121376657229092,
1.));
#8867=CARTESIAN_POINT('Origin',(5.71194030551894,18.3863276037678,1.00000000000001));
#8868=CARTESIAN_POINT('',(8.38815709466699,16.8555209332691,1.));
#8869=CARTESIAN_POINT('Origin',(13.1721719029963,14.0791608827472,1.00000000000001));
#8870=CARTESIAN_POINT('',(7.8662441728175,16.6919694958575,1.));
#8871=CARTESIAN_POINT('Origin',(8.03787131840625,17.0588061391976,1.));
#8872=CARTESIAN_POINT('Origin',(-4.48686227061401E-12,-0.121376657241696,
1.));
#8873=CARTESIAN_POINT('',(4.6751602538457,18.2285309132174,1.));
#8874=CARTESIAN_POINT('Origin',(9.93187057291089,16.5074935987231,1.00000000000001));
#8875=CARTESIAN_POINT('',(4.19865663743457,17.9600416690753,1.));
#8876=CARTESIAN_POINT('Origin',(4.29026369134224,18.3545453416492,1.));
#8877=CARTESIAN_POINT('Origin',(-1.20715069884536E-12,-0.121376657237335,
1.));
#8878=CARTESIAN_POINT('',(0.757836476023318,18.7995618797112,1.));
#8879=CARTESIAN_POINT('Origin',(6.25749884038657,18.2090648903413,1.00000000000001));
#8880=CARTESIAN_POINT('',(0.347567659605759,18.4378690971619,1.));
#8881=CARTESIAN_POINT('Origin',(0.355150953997157,18.8427980954396,1.));
#8882=CARTESIAN_POINT('',(-0.347567659605682,18.4378690971619,1.));
#8883=CARTESIAN_POINT('Origin',(3.74591850593742E-14,-0.121376657224663,
1.));
#8884=CARTESIAN_POINT('',(-0.757836476023246,18.7995618797112,1.));
#8885=CARTESIAN_POINT('Origin',(-0.355150953997079,18.8427980954396,1.));
#8886=CARTESIAN_POINT('Origin',(-6.25749884038647,18.2090648903413,1.00000000000001));
#8887=CARTESIAN_POINT('',(-3.19260839230391,18.5436570394042,1.));
#8888=CARTESIAN_POINT('Origin',(2.30964438172673,19.109507927113,1.00000000000001));
#8889=CARTESIAN_POINT('',(-3.51871169276225,18.1045684286397,1.));
#8890=CARTESIAN_POINT('Origin',(-3.5954835842407,18.5022254123315,1.));
#8891=CARTESIAN_POINT('',(-4.19865663743425,17.9600416690753,1.));
#8892=CARTESIAN_POINT('Origin',(1.46844342241437E-12,-0.121376657238497,
1.));
#8893=CARTESIAN_POINT('',(-4.67516025384538,18.2285309132174,1.));
#8894=CARTESIAN_POINT('Origin',(-4.29026369134191,18.3545453416493,1.));
#8895=CARTESIAN_POINT('Origin',(-9.93187057291062,16.5074935987233,1.00000000000001));
#8896=CARTESIAN_POINT('',(-7.0035209540528,17.4720006617854,1.));
#8897=CARTESIAN_POINT('Origin',(-1.7391526193181,19.1694690275264,1.00000000000001));
#8898=CARTESIAN_POINT('',(-7.23120645950465,16.9747065020771,1.));
#8899=CARTESIAN_POINT('Origin',(-7.38897823680293,17.3477119528257,1.));
#8900=CARTESIAN_POINT('',(-7.8662441728172,16.6919694958576,1.));
#8901=CARTESIAN_POINT('Origin',(5.46524631106493E-12,-0.12137665724324,
1.));
#8902=CARTESIAN_POINT('',(-8.38815709466669,16.8555209332692,1.));
#8903=CARTESIAN_POINT('Origin',(-8.03787131840593,17.0588061391977,1.));
#8904=CARTESIAN_POINT('Origin',(-13.1721719029961,14.0791608827473,1.00000000000001));
#8905=CARTESIAN_POINT('',(-10.5083460434875,15.6314292729347,1.));
#8906=CARTESIAN_POINT('Origin',(-5.71194030551858,18.3863276037679,1.00000000000001));
#8907=CARTESIAN_POINT('',(-10.6276628047883,15.0976637053439,1.));
#8908=CARTESIAN_POINT('Origin',(-10.8595390841655,15.4297154950728,1.));
#8909=CARTESIAN_POINT('',(-11.1900390914206,14.6890734163638,1.));
#8910=CARTESIAN_POINT('Origin',(-9.26342336171615E-13,-0.121376657230733,
1.));
#8911=CARTESIAN_POINT('',(-11.7345512196076,14.7405390644231,1.));
#8912=CARTESIAN_POINT('Origin',(-11.4341853988698,15.0122105088786,1.));
#8913=CARTESIAN_POINT('Origin',(-15.8367861138271,11.030196534535,1.00000000000001));
#8914=CARTESIAN_POINT('',(-13.5539059861829,13.1023846745862,1.));
#8915=CARTESIAN_POINT('Origin',(-9.43508879143725,16.7943106939854,1.00000000000001));
#8916=CARTESIAN_POINT('',(-13.5596392883185,12.555475815708,1.));
#8917=CARTESIAN_POINT('Origin',(-13.8554859637,12.8320616878448,1.));
#8918=CARTESIAN_POINT('',(-14.0247756059639,12.0388896002294,1.));
#8919=CARTESIAN_POINT('Origin',(1.06442632485937E-11,-0.1213766572417,1.));
#8920=CARTESIAN_POINT('',(-14.5680891476275,11.9760201631568,1.));
#8921=CARTESIAN_POINT('Origin',(-14.330770710094,12.3042045003922,1.));
#8922=CARTESIAN_POINT('Origin',(-17.8092567781527,7.49385492665735,1.00000000000001));
#8923=CARTESIAN_POINT('',(-16.0070951984252,9.99539825139022,1.));
#8924=CARTESIAN_POINT('Origin',(-12.745878622591,14.4629970764811,1.00000000000001));
#8925=CARTESIAN_POINT('',(-15.8989944685809,9.45924864271742,1.));
#8926=CARTESIAN_POINT('Origin',(-16.2458816206226,9.66828046744359,1.));
#8927=CARTESIAN_POINT('',(-16.2465621281866,8.85724379721251,1.));
#8928=CARTESIAN_POINT('Origin',(3.8372083288607E-12,-0.121376657234332,
1.));
#8929=CARTESIAN_POINT('',(-16.7649316744485,8.68278697108894,1.));
#8930=CARTESIAN_POINT('Origin',(-16.6010325746197,9.05314097076402,1.));
#8931=CARTESIAN_POINT('Origin',(-19.0033774629776,3.6246911566283,1.));
#8932=CARTESIAN_POINT('',(-17.7606975399316,6.44626021901535,1.));
#8933=CARTESIAN_POINT('Origin',(-15.4996123964262,11.4942763432236,1.00000000000001));
#8934=CARTESIAN_POINT('',(-17.5434872987263,5.94430217117825,1.));
#8935=CARTESIAN_POINT('Origin',(-17.9262542943349,6.0766442547072,1.));
#8936=CARTESIAN_POINT('',(-17.7582959257529,5.2831891961353,1.));
#8937=CARTESIAN_POINT('Origin',(7.0082828429463E-13,-0.121376657232305,
1.));
#8938=CARTESIAN_POINT('',(-18.2290662400284,5.00476958139915,1.));
#8939=CARTESIAN_POINT('Origin',(-18.1457496550421,5.40110699657241,1.));
#8940=CARTESIAN_POINT('Origin',(-19.3669593643481,-0.408193752494226,1.00000000000001));
#8941=CARTESIAN_POINT('',(-18.7380721736606,2.61008494013019,1.));
#8942=CARTESIAN_POINT('Origin',(-17.5759387331454,8.01789583575926,1.00000000000001));
#8943=CARTESIAN_POINT('',(-18.4212455509255,2.16425642848123,1.));
#8944=CARTESIAN_POINT('Origin',(-18.8231636356729,2.21412478671497,1.));
#8945=CARTESIAN_POINT('',(-18.4939069776057,1.47292913328164,1.));
#8946=CARTESIAN_POINT('Origin',(-3.32199545649559E-12,-0.121376657231894,
1.));
#8947=CARTESIAN_POINT('',(-18.8965031381544,1.10271500310242,1.));
#8948=CARTESIAN_POINT('Origin',(-18.8974104025716,1.50771398689285,1.));
#8949=CARTESIAN_POINT('Origin',(-18.8841122085149,-4.42854337825269,1.00000000000001));
#8950=CARTESIAN_POINT('',(-18.8965031381544,-1.34546831756664,1.));
#8951=CARTESIAN_POINT('Origin',(-18.8841122085148,4.18579006378843,1.00000000000001));
#8952=CARTESIAN_POINT('',(-18.4939069776057,-1.71568244774586,1.));
#8953=CARTESIAN_POINT('Origin',(-18.8974104025717,-1.75046730135707,1.));
#8954=CARTESIAN_POINT('',(-18.4212455509255,-2.40700974294545,1.));
#8955=CARTESIAN_POINT('Origin',(3.52669282666085E-12,-0.121376657231728,
1.));
#8956=CARTESIAN_POINT('',(-18.7380721736606,-2.85283825459442,1.));
#8957=CARTESIAN_POINT('Origin',(-18.8231636356729,-2.45687810117919,1.));
#8958=CARTESIAN_POINT('Origin',(-17.5759387331454,-8.26064915022349,1.00000000000001));
#8959=CARTESIAN_POINT('',(-18.2290662400285,-5.24752289586338,1.));
#8960=CARTESIAN_POINT('Origin',(-19.3669593643481,0.16544043803,1.00000000000001));
#8961=CARTESIAN_POINT('',(-17.758295925753,-5.52594251059953,1.));
#8962=CARTESIAN_POINT('Origin',(-18.1457496550421,-5.64386031103663,1.));
#8963=CARTESIAN_POINT('',(-17.5434872987264,-6.18705548564248,1.));
#8964=CARTESIAN_POINT('Origin',(9.73179870022989E-13,-0.121376657231793,
1.));
#8965=CARTESIAN_POINT('',(-17.7606975399316,-6.68901353347958,1.));
#8966=CARTESIAN_POINT('Origin',(-17.926254294335,-6.31939756917143,1.));
#8967=CARTESIAN_POINT('Origin',(-15.4996123964263,-11.7370296576879,1.));
#8968=CARTESIAN_POINT('',(-16.7649316744485,-8.92554028555318,1.));
#8969=CARTESIAN_POINT('Origin',(-19.0033774629776,-3.86744447109251,1.00000000000001));
#8970=CARTESIAN_POINT('',(-16.2465621281866,-9.09999711167674,1.));
#8971=CARTESIAN_POINT('Origin',(-16.6010325746198,-9.29589428522826,1.));
#8972=CARTESIAN_POINT('',(-15.8989944685809,-9.70200195718166,1.));
#8973=CARTESIAN_POINT('Origin',(-2.48412401759879E-12,-0.121376657233779,
1.));
#8974=CARTESIAN_POINT('',(-16.0070951984253,-10.2381515658545,1.));
#8975=CARTESIAN_POINT('Origin',(-16.2458816206227,-9.91103378190783,1.));
#8976=CARTESIAN_POINT('Origin',(-12.7458786225912,-14.7057503909453,1.00000000000001));
#8977=CARTESIAN_POINT('',(-14.5680891476276,-12.218773477621,1.));
#8978=CARTESIAN_POINT('Origin',(-17.8092567781527,-7.73660824112161,1.));
#8979=CARTESIAN_POINT('',(-14.024775605964,-12.2816429146937,1.));
#8980=CARTESIAN_POINT('Origin',(-14.3307707100941,-12.5469578148565,1.));
#8981=CARTESIAN_POINT('',(-13.5596392883186,-12.7982291301722,1.));
#8982=CARTESIAN_POINT('Origin',(-8.74300631892311E-13,-0.121376657233123,
1.));
#8983=CARTESIAN_POINT('Origin',(-13.8554859637001,-13.0748150023091,1.));
#8984=CARTESIAN_POINT('',(-1.49999999999993,5.62862334276781,1.));
#8985=CARTESIAN_POINT('',(-1.49999999999993,5.62862334276781,1.));
#8986=CARTESIAN_POINT('',(1.49999999999993,5.62862334276781,1.));
#8987=CARTESIAN_POINT('',(-1.49999999999993,5.62862334276781,1.));
#8988=CARTESIAN_POINT('',(1.49999999999993,5.62862334276781,1.));
#8989=CARTESIAN_POINT('Origin',(3.64291929955129E-14,-0.121376657232174,
1.));
#8990=CARTESIAN_POINT('',(1.74510424621309,-21.650766132316,4.082419099807E-15));
#8991=CARTESIAN_POINT('Origin',(-6.25749884038648,-18.4518182048057,-0.999999999999996));
#8992=CARTESIAN_POINT('',(-0.757836476023246,-19.0423151941755,-0.999999999999996));
#8993=CARTESIAN_POINT('Origin',(6.25749884038655,-18.4518182048057,-0.999999999999996));
#8994=CARTESIAN_POINT('',(0.757836476023317,-19.0423151941755,-0.999999999999996));
#8995=CARTESIAN_POINT('Origin',(3.64291929955129E-14,-0.121376657232175,
-0.999999999999996));
#8996=CARTESIAN_POINT('',(-0.347567659605688,-18.6806224116263,-0.999999999999996));
#8997=CARTESIAN_POINT('',(0.347567659605753,-18.6806224116263,-0.999999999999996));
#8998=CARTESIAN_POINT('Origin',(-0.355150953997086,-19.085551409904,-0.999999999999996));
#8999=CARTESIAN_POINT('Origin',(0.355150953997151,-19.085551409904,-0.999999999999996));
#9000=CARTESIAN_POINT('Origin',(2.30964438172655,-19.3522612415774,-0.999999999999996));
#9001=CARTESIAN_POINT('',(-3.19260839230403,-18.7864103538685,-0.999999999999996));
#9002=CARTESIAN_POINT('Origin',(-9.93187057291073,-16.7502469131875,-0.999999999999996));
#9003=CARTESIAN_POINT('',(-4.6751602538455,-18.4712842276817,-0.999999999999996));
#9004=CARTESIAN_POINT('Origin',(-4.29026369134204,-18.5972986561136,-0.999999999999996));
#9005=CARTESIAN_POINT('',(-4.19865663743438,-18.2027949835397,-0.999999999999996));
#9006=CARTESIAN_POINT('Origin',(3.64291929955129E-14,-0.121376657232175,
-0.999999999999996));
#9007=CARTESIAN_POINT('',(-3.51871169276238,-18.3473217431041,-0.999999999999996));
#9008=CARTESIAN_POINT('Origin',(-3.59548358424083,-18.7449787267958,-0.999999999999996));
#9009=CARTESIAN_POINT('Origin',(15.4996123964264,11.4942763432235,-0.999999999999996));
#9010=CARTESIAN_POINT('Origin',(19.3669593643482,-0.408193752494492,-0.999999999999996));
#9011=CARTESIAN_POINT('',(18.2290662400286,5.0047695813989,-0.999999999999996));
#9012=CARTESIAN_POINT('Origin',(18.1457496550422,5.40110699657215,-0.999999999999996));
#9013=CARTESIAN_POINT('',(17.7582959257531,5.28318919613505,-0.999999999999996));
#9014=CARTESIAN_POINT('Origin',(3.64291929955129E-14,-0.121376657232175,
-0.999999999999996));
#9015=CARTESIAN_POINT('Origin',(12.7458786225913,14.4629970764809,-0.999999999999996));
#9016=CARTESIAN_POINT('Origin',(19.0033774629777,3.62469115662802,-0.999999999999996));
#9017=CARTESIAN_POINT('',(16.7649316744487,8.68278697108871,-0.999999999999996));
#9018=CARTESIAN_POINT('Origin',(16.6010325746199,9.05314097076379,-0.999999999999996));
#9019=CARTESIAN_POINT('',(16.2465621281868,8.85724379721227,-0.999999999999996));
#9020=CARTESIAN_POINT('Origin',(3.64291929955129E-14,-0.121376657232175,
-0.999999999999996));
#9021=CARTESIAN_POINT('Origin',(5.71194030551891,18.3863276037678,-0.999999999999996));
#9022=CARTESIAN_POINT('Origin',(15.8367861138273,11.0301965345348,-0.999999999999996));
#9023=CARTESIAN_POINT('',(11.7345512196078,14.740539064423,-0.999999999999996));
#9024=CARTESIAN_POINT('Origin',(11.4341853988701,15.0122105088784,-0.999999999999996));
#9025=CARTESIAN_POINT('',(11.1900390914209,14.6890734163636,-0.999999999999996));
#9026=CARTESIAN_POINT('Origin',(3.64291929955129E-14,-0.121376657232175,
-0.999999999999996));
#9027=CARTESIAN_POINT('Origin',(9.4350887914376,16.7943106939853,-0.999999999999996));
#9028=CARTESIAN_POINT('Origin',(17.8092567781529,7.49385492665712,-0.999999999999996));
#9029=CARTESIAN_POINT('',(14.5680891476277,11.9760201631566,-0.999999999999996));
#9030=CARTESIAN_POINT('Origin',(14.3307707100943,12.304204500392,-0.999999999999996));
#9031=CARTESIAN_POINT('',(14.0247756059641,12.0388896002292,-0.999999999999996));
#9032=CARTESIAN_POINT('Origin',(3.64291929955129E-14,-0.121376657232175,
-0.999999999999996));
#9033=CARTESIAN_POINT('Origin',(17.5759387331456,8.01789583575903,-0.999999999999996));
#9034=CARTESIAN_POINT('Origin',(18.8841122085149,-4.42854337825292,-0.999999999999996));
#9035=CARTESIAN_POINT('',(18.8965031381544,1.10271500310216,-0.999999999999996));
#9036=CARTESIAN_POINT('Origin',(18.8974104025717,1.50771398689258,-0.999999999999996));
#9037=CARTESIAN_POINT('',(18.4939069776058,1.47292913328138,-0.999999999999996));
#9038=CARTESIAN_POINT('Origin',(3.64291929955129E-14,-0.121376657232175,
-0.999999999999996));
#9039=CARTESIAN_POINT('Origin',(18.884112208515,4.18579006378819,-0.999999999999996));
#9040=CARTESIAN_POINT('',(18.8965031381544,-1.34546831756689,-0.999999999999996));
#9041=CARTESIAN_POINT('Origin',(17.5759387331454,-8.26064915022373,-0.999999999999996));
#9042=CARTESIAN_POINT('Origin',(3.64291929955129E-14,-0.121376657232175,
-0.999999999999996));
#9043=CARTESIAN_POINT('',(18.4939069776058,-1.71568244774611,-0.999999999999996));
#9044=CARTESIAN_POINT('Origin',(18.8974104025717,-1.75046730135732,-0.999999999999996));
#9045=CARTESIAN_POINT('Origin',(19.3669593643482,0.165440438029751,-0.999999999999996));
#9046=CARTESIAN_POINT('',(18.2290662400285,-5.24752289586362,-0.999999999999996));
#9047=CARTESIAN_POINT('Origin',(15.4996123964262,-11.7370296576881,-0.999999999999996));
#9048=CARTESIAN_POINT('Origin',(3.64291929955129E-14,-0.121376657232175,
-0.999999999999996));
#9049=CARTESIAN_POINT('',(17.758295925753,-5.52594251059977,-0.999999999999996));
#9050=CARTESIAN_POINT('Origin',(18.1457496550421,-5.64386031103687,-0.999999999999996));
#9051=CARTESIAN_POINT('Origin',(19.0033774629777,-3.86744447109277,-0.999999999999996));
#9052=CARTESIAN_POINT('',(16.7649316744485,-8.92554028555341,-0.999999999999996));
#9053=CARTESIAN_POINT('Origin',(12.745878622591,-14.7057503909455,-0.999999999999996));
#9054=CARTESIAN_POINT('Origin',(3.64291929955129E-14,-0.121376657232175,
-0.999999999999996));
#9055=CARTESIAN_POINT('',(16.2465621281866,-9.09999711167697,-0.999999999999996));
#9056=CARTESIAN_POINT('Origin',(16.6010325746197,-9.29589428522849,-0.999999999999996));
#9057=CARTESIAN_POINT('Origin',(15.836786113827,-11.2729498489995,-0.999999999999996));
#9058=CARTESIAN_POINT('',(11.7345512196075,-14.9832923788876,-0.999999999999996));
#9059=CARTESIAN_POINT('Origin',(5.71194030551853,-18.6290809182323,-0.999999999999996));
#9060=CARTESIAN_POINT('Origin',(3.64291929955129E-14,-0.121376657232175,
-0.999999999999996));
#9061=CARTESIAN_POINT('',(11.1900390914206,-14.9318267308282,-0.999999999999996));
#9062=CARTESIAN_POINT('Origin',(11.4341853988697,-15.254963823343,-0.999999999999996));
#9063=CARTESIAN_POINT('Origin',(17.8092567781527,-7.73660824112183,-0.999999999999996));
#9064=CARTESIAN_POINT('',(14.5680891476275,-12.2187734776212,-0.999999999999996));
#9065=CARTESIAN_POINT('Origin',(9.43508879143726,-17.0370640084498,-0.999999999999996));
#9066=CARTESIAN_POINT('Origin',(3.64291929955129E-14,-0.121376657232175,
-0.999999999999996));
#9067=CARTESIAN_POINT('',(14.0247756059639,-12.2816429146939,-0.999999999999996));
#9068=CARTESIAN_POINT('Origin',(14.330770710094,-12.5469578148567,-0.999999999999996));
#9069=CARTESIAN_POINT('Origin',(13.172171902996,-14.3219141972118,-0.999999999999996));
#9070=CARTESIAN_POINT('',(8.38815709466665,-17.0982742477336,-0.999999999999996));
#9071=CARTESIAN_POINT('Origin',(3.64291929955129E-14,-0.121376657232175,
-0.999999999999996));
#9072=CARTESIAN_POINT('',(7.86624417281716,-16.934722810322,-0.999999999999996));
#9073=CARTESIAN_POINT('Origin',(8.0378713184059,-17.3015594536621,-0.999999999999996));
#9074=CARTESIAN_POINT('Origin',(9.93187057291058,-16.7502469131877,-0.999999999999996));
#9075=CARTESIAN_POINT('',(4.67516025384533,-18.4712842276818,-0.999999999999996));
#9076=CARTESIAN_POINT('Origin',(3.64291929955129E-14,-0.121376657232175,
-0.999999999999996));
#9077=CARTESIAN_POINT('',(4.1986566374342,-18.2027949835397,-0.999999999999996));
#9078=CARTESIAN_POINT('Origin',(4.29026369134186,-18.5972986561137,-0.999999999999996));
#9079=CARTESIAN_POINT('Origin',(13.1721719029963,14.0791608827472,-0.999999999999996));
#9080=CARTESIAN_POINT('',(8.38815709466699,16.8555209332691,-0.999999999999996));
#9081=CARTESIAN_POINT('Origin',(8.03787131840625,17.0588061391976,-0.999999999999996));
#9082=CARTESIAN_POINT('',(7.8662441728175,16.6919694958575,-0.999999999999996));
#9083=CARTESIAN_POINT('Origin',(3.64291929955129E-14,-0.121376657232175,
-0.999999999999996));
#9084=CARTESIAN_POINT('Origin',(9.93187057291091,16.5074935987231,-0.999999999999996));
#9085=CARTESIAN_POINT('',(4.6751602538457,18.2285309132174,-0.999999999999996));
#9086=CARTESIAN_POINT('Origin',(4.29026369134223,18.3545453416492,-0.999999999999996));
#9087=CARTESIAN_POINT('',(4.19865663743457,17.9600416690753,-0.999999999999996));
#9088=CARTESIAN_POINT('Origin',(3.64291929955129E-14,-0.121376657232175,
-0.999999999999996));
#9089=CARTESIAN_POINT('Origin',(-6.25749884038648,18.2090648903413,-0.999999999999996));
#9090=CARTESIAN_POINT('',(-0.757836476023246,18.7995618797112,-0.999999999999996));
#9091=CARTESIAN_POINT('Origin',(6.25749884038655,18.2090648903413,-0.999999999999996));
#9092=CARTESIAN_POINT('',(0.757836476023318,18.7995618797112,-0.999999999999996));
#9093=CARTESIAN_POINT('Origin',(0.355150953997157,18.8427980954396,-0.999999999999996));
#9094=CARTESIAN_POINT('',(0.347567659605759,18.4378690971619,-0.999999999999996));
#9095=CARTESIAN_POINT('Origin',(3.64291929955129E-14,-0.121376657232175,
-0.999999999999996));
#9096=CARTESIAN_POINT('',(-0.347567659605682,18.4378690971619,-0.999999999999996));
#9097=CARTESIAN_POINT('Origin',(-0.355150953997079,18.8427980954396,-0.999999999999996));
#9098=CARTESIAN_POINT('Origin',(-9.93187057291061,16.5074935987233,-0.999999999999996));
#9099=CARTESIAN_POINT('',(-4.67516025384538,18.2285309132174,-0.999999999999996));
#9100=CARTESIAN_POINT('Origin',(2.30964438172668,19.109507927113,-0.999999999999996));
#9101=CARTESIAN_POINT('',(-3.19260839230391,18.5436570394042,-0.999999999999996));
#9102=CARTESIAN_POINT('Origin',(-3.5954835842407,18.5022254123315,-0.999999999999996));
#9103=CARTESIAN_POINT('',(-3.51871169276225,18.1045684286397,-0.999999999999996));
#9104=CARTESIAN_POINT('Origin',(3.64291929955129E-14,-0.121376657232175,
-0.999999999999996));
#9105=CARTESIAN_POINT('',(-4.19865663743425,17.9600416690753,-0.999999999999996));
#9106=CARTESIAN_POINT('Origin',(-4.29026369134191,18.3545453416493,-0.999999999999996));
#9107=CARTESIAN_POINT('Origin',(-17.8092567781527,7.49385492665736,-0.999999999999996));
#9108=CARTESIAN_POINT('',(-14.5680891476275,11.9760201631568,-0.999999999999996));
#9109=CARTESIAN_POINT('Origin',(-9.4350887914373,16.7943106939854,-0.999999999999996));
#9110=CARTESIAN_POINT('',(-13.5539059861829,13.1023846745862,-0.999999999999996));
#9111=CARTESIAN_POINT('Origin',(-13.8554859637,12.8320616878448,-0.999999999999996));
#9112=CARTESIAN_POINT('',(-13.5596392883185,12.555475815708,-0.999999999999996));
#9113=CARTESIAN_POINT('Origin',(3.64291929955129E-14,-0.121376657232175,
-0.999999999999996));
#9114=CARTESIAN_POINT('',(-14.0247756059639,12.0388896002294,-0.999999999999996));
#9115=CARTESIAN_POINT('Origin',(-14.330770710094,12.3042045003922,-0.999999999999996));
#9116=CARTESIAN_POINT('Origin',(-19.0033774629776,3.62469115662829,-0.999999999999996));
#9117=CARTESIAN_POINT('',(-16.7649316744485,8.68278697108894,-0.999999999999996));
#9118=CARTESIAN_POINT('Origin',(-12.7458786225911,14.462997076481,-0.999999999999996));
#9119=CARTESIAN_POINT('',(-16.0070951984252,9.99539825139022,-0.999999999999996));
#9120=CARTESIAN_POINT('Origin',(-16.2458816206226,9.66828046744359,-0.999999999999996));
#9121=CARTESIAN_POINT('',(-15.8989944685809,9.45924864271742,-0.999999999999996));
#9122=CARTESIAN_POINT('Origin',(3.64291929955129E-14,-0.121376657232175,
-0.999999999999996));
#9123=CARTESIAN_POINT('',(-16.2465621281866,8.85724379721251,-0.999999999999996));
#9124=CARTESIAN_POINT('Origin',(-16.6010325746197,9.05314097076402,-0.999999999999996));
#9125=CARTESIAN_POINT('Origin',(-15.8367861138271,11.0301965345351,-0.999999999999996));
#9126=CARTESIAN_POINT('',(-11.7345512196076,14.7405390644231,-0.999999999999996));
#9127=CARTESIAN_POINT('Origin',(-5.71194030551859,18.3863276037679,-0.999999999999996));
#9128=CARTESIAN_POINT('',(-10.5083460434875,15.6314292729347,-0.999999999999996));
#9129=CARTESIAN_POINT('Origin',(-10.8595390841655,15.4297154950728,-0.999999999999996));
#9130=CARTESIAN_POINT('',(-10.6276628047883,15.0976637053439,-0.999999999999996));
#9131=CARTESIAN_POINT('Origin',(3.64291929955129E-14,-0.121376657232175,
-0.999999999999996));
#9132=CARTESIAN_POINT('',(-11.1900390914206,14.6890734163638,-0.999999999999996));
#9133=CARTESIAN_POINT('Origin',(-11.4341853988698,15.0122105088786,-0.999999999999996));
#9134=CARTESIAN_POINT('Origin',(-13.1721719029961,14.0791608827474,-0.999999999999996));
#9135=CARTESIAN_POINT('',(-8.38815709466669,16.8555209332692,-0.999999999999996));
#9136=CARTESIAN_POINT('Origin',(-1.73915261931814,19.1694690275264,-0.999999999999996));
#9137=CARTESIAN_POINT('',(-7.0035209540528,17.4720006617854,-0.999999999999996));
#9138=CARTESIAN_POINT('Origin',(-7.38897823680293,17.3477119528256,-0.999999999999996));
#9139=CARTESIAN_POINT('',(-7.23120645950465,16.9747065020771,-0.999999999999996));
#9140=CARTESIAN_POINT('Origin',(3.64291929955129E-14,-0.121376657232175,
-0.999999999999996));
#9141=CARTESIAN_POINT('',(-7.8662441728172,16.6919694958576,-0.999999999999996));
#9142=CARTESIAN_POINT('Origin',(-8.03787131840594,17.0588061391977,-0.999999999999996));
#9143=CARTESIAN_POINT('Origin',(-19.3669593643481,-0.408193752494226,-0.999999999999996));
#9144=CARTESIAN_POINT('',(-18.2290662400284,5.00476958139915,-0.999999999999996));
#9145=CARTESIAN_POINT('Origin',(-15.4996123964262,11.4942763432237,-0.999999999999996));
#9146=CARTESIAN_POINT('',(-17.7606975399316,6.44626021901535,-0.999999999999996));
#9147=CARTESIAN_POINT('Origin',(-17.9262542943349,6.0766442547072,-0.999999999999996));
#9148=CARTESIAN_POINT('',(-17.5434872987263,5.94430217117825,-0.999999999999996));
#9149=CARTESIAN_POINT('Origin',(3.64291929955129E-14,-0.121376657232175,
-0.999999999999996));
#9150=CARTESIAN_POINT('',(-17.7582959257529,5.2831891961353,-0.999999999999996));
#9151=CARTESIAN_POINT('Origin',(-18.1457496550421,5.40110699657241,-0.999999999999996));
#9152=CARTESIAN_POINT('Origin',(-18.8841122085149,-4.42854337825267,-0.999999999999996));
#9153=CARTESIAN_POINT('',(-18.8965031381544,1.10271500310242,-0.999999999999996));
#9154=CARTESIAN_POINT('Origin',(-17.5759387331454,8.01789583575926,-0.999999999999996));
#9155=CARTESIAN_POINT('',(-18.7380721736606,2.61008494013019,-0.999999999999996));
#9156=CARTESIAN_POINT('Origin',(-18.8231636356729,2.21412478671498,-0.999999999999996));
#9157=CARTESIAN_POINT('',(-18.4212455509255,2.16425642848123,-0.999999999999996));
#9158=CARTESIAN_POINT('Origin',(3.64291929955129E-14,-0.121376657232175,
-0.999999999999996));
#9159=CARTESIAN_POINT('',(-18.4939069776057,1.47292913328164,-0.999999999999996));
#9160=CARTESIAN_POINT('Origin',(-18.8974104025716,1.50771398689285,-0.999999999999996));
#9161=CARTESIAN_POINT('Origin',(-17.5759387331454,-8.2606491502235,-0.999999999999996));
#9162=CARTESIAN_POINT('',(-18.7380721736606,-2.85283825459442,-0.999999999999996));
#9163=CARTESIAN_POINT('Origin',(-18.8841122085148,4.18579006378844,-0.999999999999996));
#9164=CARTESIAN_POINT('',(-18.8965031381544,-1.34546831756664,-0.999999999999996));
#9165=CARTESIAN_POINT('Origin',(-18.8974104025717,-1.75046730135707,-0.999999999999996));
#9166=CARTESIAN_POINT('',(-18.4939069776057,-1.71568244774586,-0.999999999999996));
#9167=CARTESIAN_POINT('Origin',(3.64291929955129E-14,-0.121376657232175,
-0.999999999999996));
#9168=CARTESIAN_POINT('',(-18.4212455509255,-2.40700974294545,-0.999999999999996));
#9169=CARTESIAN_POINT('Origin',(-18.8231636356729,-2.4568781011792,-0.999999999999996));
#9170=CARTESIAN_POINT('Origin',(-15.4996123964263,-11.7370296576879,-0.999999999999996));
#9171=CARTESIAN_POINT('',(-17.7606975399316,-6.68901353347958,-0.999999999999996));
#9172=CARTESIAN_POINT('Origin',(-19.3669593643481,0.165440438030005,-0.999999999999996));
#9173=CARTESIAN_POINT('',(-18.2290662400285,-5.24752289586338,-0.999999999999996));
#9174=CARTESIAN_POINT('Origin',(-18.1457496550421,-5.64386031103663,-0.999999999999996));
#9175=CARTESIAN_POINT('',(-17.758295925753,-5.52594251059953,-0.999999999999996));
#9176=CARTESIAN_POINT('Origin',(3.64291929955129E-14,-0.121376657232175,
-0.999999999999996));
#9177=CARTESIAN_POINT('',(-17.5434872987264,-6.18705548564248,-0.999999999999996));
#9178=CARTESIAN_POINT('Origin',(-17.926254294335,-6.31939756917143,-0.999999999999996));
#9179=CARTESIAN_POINT('Origin',(-1.73915261931827,-19.4122223419907,-0.999999999999996));
#9180=CARTESIAN_POINT('',(-7.00352095405292,-17.7147539762497,-0.999999999999996));
#9181=CARTESIAN_POINT('Origin',(-13.1721719029961,-14.3219141972116,-0.999999999999996));
#9182=CARTESIAN_POINT('',(-8.38815709466681,-17.0982742477335,-0.999999999999996));
#9183=CARTESIAN_POINT('Origin',(-8.03787131840606,-17.301559453662,-0.999999999999996));
#9184=CARTESIAN_POINT('',(-7.86624417281732,-16.9347228103219,-0.999999999999996));
#9185=CARTESIAN_POINT('Origin',(3.64291929955129E-14,-0.121376657232175,
-0.999999999999996));
#9186=CARTESIAN_POINT('',(-7.23120645950477,-17.2174598165414,-0.999999999999996));
#9187=CARTESIAN_POINT('Origin',(-7.38897823680305,-17.5904652672899,-0.999999999999996));
#9188=CARTESIAN_POINT('Origin',(-5.71194030551871,-18.6290809182322,-0.999999999999996));
#9189=CARTESIAN_POINT('',(-10.5083460434876,-15.874182587399,-0.999999999999996));
#9190=CARTESIAN_POINT('Origin',(-15.8367861138271,-11.2729498489993,-0.999999999999996));
#9191=CARTESIAN_POINT('',(-11.7345512196077,-14.9832923788874,-0.999999999999996));
#9192=CARTESIAN_POINT('Origin',(-11.4341853988699,-15.2549638233429,-0.999999999999996));
#9193=CARTESIAN_POINT('',(-11.1900390914207,-14.931826730828,-0.999999999999996));
#9194=CARTESIAN_POINT('Origin',(3.64291929955129E-14,-0.121376657232175,
-0.999999999999996));
#9195=CARTESIAN_POINT('',(-10.6276628047884,-15.3404170198082,-0.999999999999996));
#9196=CARTESIAN_POINT('Origin',(-10.8595390841656,-15.6724688095371,-0.999999999999996));
#9197=CARTESIAN_POINT('Origin',(-12.7458786225912,-14.7057503909453,-0.999999999999996));
#9198=CARTESIAN_POINT('',(-16.0070951984253,-10.2381515658545,-0.999999999999996));
#9199=CARTESIAN_POINT('Origin',(-19.0033774629776,-3.86744447109251,-0.999999999999996));
#9200=CARTESIAN_POINT('',(-16.7649316744485,-8.92554028555318,-0.999999999999996));
#9201=CARTESIAN_POINT('Origin',(-16.6010325746198,-9.29589428522826,-0.999999999999996));
#9202=CARTESIAN_POINT('',(-16.2465621281866,-9.09999711167674,-0.999999999999996));
#9203=CARTESIAN_POINT('Origin',(3.64291929955129E-14,-0.121376657232175,
-0.999999999999996));
#9204=CARTESIAN_POINT('',(-15.8989944685809,-9.70200195718166,-0.999999999999996));
#9205=CARTESIAN_POINT('Origin',(-16.2458816206227,-9.91103378190782,-0.999999999999996));
#9206=CARTESIAN_POINT('Origin',(-9.43508879143742,-17.0370640084497,-0.999999999999996));
#9207=CARTESIAN_POINT('',(-13.5539059861829,-13.3451379890505,-0.999999999999996));
#9208=CARTESIAN_POINT('Origin',(-17.8092567781528,-7.73660824112159,-0.999999999999996));
#9209=CARTESIAN_POINT('',(-14.5680891476276,-12.218773477621,-0.999999999999996));
#9210=CARTESIAN_POINT('Origin',(-14.3307707100941,-12.5469578148565,-0.999999999999996));
#9211=CARTESIAN_POINT('',(-14.024775605964,-12.2816429146937,-0.999999999999996));
#9212=CARTESIAN_POINT('Origin',(3.64291929955129E-14,-0.121376657232175,
-0.999999999999996));
#9213=CARTESIAN_POINT('',(-13.5596392883186,-12.7982291301722,-0.999999999999996));
#9214=CARTESIAN_POINT('Origin',(-13.8554859637001,-13.0748150023091,-0.999999999999996));
#9215=CARTESIAN_POINT('Origin',(-1.49999999999993,5.62862334276781,-4.));
#9216=CARTESIAN_POINT('',(1.49999999999993,5.62862334276781,-4.));
#9217=CARTESIAN_POINT('',(-1.49999999999993,5.62862334276781,-4.));
#9218=CARTESIAN_POINT('Origin',(-1.49999999999993,5.62862334276781,-4.));
#9219=CARTESIAN_POINT('Origin',(1.49999999999993,5.62862334276781,-4.));
#10397=UNCERTAINTY_MEASURE_WITH_UNIT(LENGTH_MEASURE(0.01),#10414,
'DISTANCE_ACCURACY_VALUE',
'Maximum model space distance between geometric entities at asserted c
onnectivities');
#10403=UNCERTAINTY_MEASURE_WITH_UNIT(LENGTH_MEASURE(0.01),#10414,
'DISTANCE_ACCURACY_VALUE',
'Maximum model space distance between geometric entities at asserted c
onnectivities');
#10407=(
GEOMETRIC_REPRESENTATION_CONTEXT(3)
GLOBAL_UNCERTAINTY_ASSIGNED_CONTEXT((#10397))
GLOBAL_UNIT_ASSIGNED_CONTEXT((#10414,#10416,#10417))
REPRESENTATION_CONTEXT('','3D')
);
#10413=(
GEOMETRIC_REPRESENTATION_CONTEXT(3)
GLOBAL_UNCERTAINTY_ASSIGNED_CONTEXT((#10403))
GLOBAL_UNIT_ASSIGNED_CONTEXT((#10414,#10416,#10417))
REPRESENTATION_CONTEXT('','3D')
);
#10414=(
LENGTH_UNIT()
NAMED_UNIT(*)
SI_UNIT(.MILLI.,.METRE.)
);
#10416=(
NAMED_UNIT(*)
PLANE_ANGLE_UNIT()
SI_UNIT($,.RADIAN.)
);
#10417=(
NAMED_UNIT(*)
SI_UNIT($,.STERADIAN.)
SOLID_ANGLE_UNIT()
);
#10421=SHAPE_DEFINITION_REPRESENTATION(#10430,#10455);
#10430=PRODUCT_DEFINITION_SHAPE('',$,#10465);
#10455=SHAPE_REPRESENTATION('',(#5466),#10407);
#10461=PRODUCT_DEFINITION_CONTEXT('part definition',#10490,'design');
#10465=PRODUCT_DEFINITION('Spur Gear','Spur Gear',#10474,#10461);
#10474=PRODUCT_DEFINITION_FORMATION('',$,#10495);
#10490=APPLICATION_CONTEXT(
'Core Data for Automotive Mechanical Design Process');
#10491=PRODUCT_CONTEXT('part definition',#10490,'mechanical');
#10495=PRODUCT('Spur Gear','Spur Gear',$,(#10491));
#10502=PRESENTATION_STYLE_ASSIGNMENT((#10506));
#10506=SURFACE_STYLE_USAGE(.BOTH.,#10510);
#10510=SURFACE_SIDE_STYLE('',(#10514));
#10514=SURFACE_STYLE_FILL_AREA(#10518);
#10518=FILL_AREA_STYLE('Opaque(61,176,222)',(#10522));
#10522=FILL_AREA_STYLE_COLOUR('Opaque(61,176,222)',#10526);
#10526=COLOUR_RGB('Opaque(61,176,222)',0.23921568627451,0.690196078431373,
0.870588235294118);
ENDSEC;
END-ISO-10303-21;
